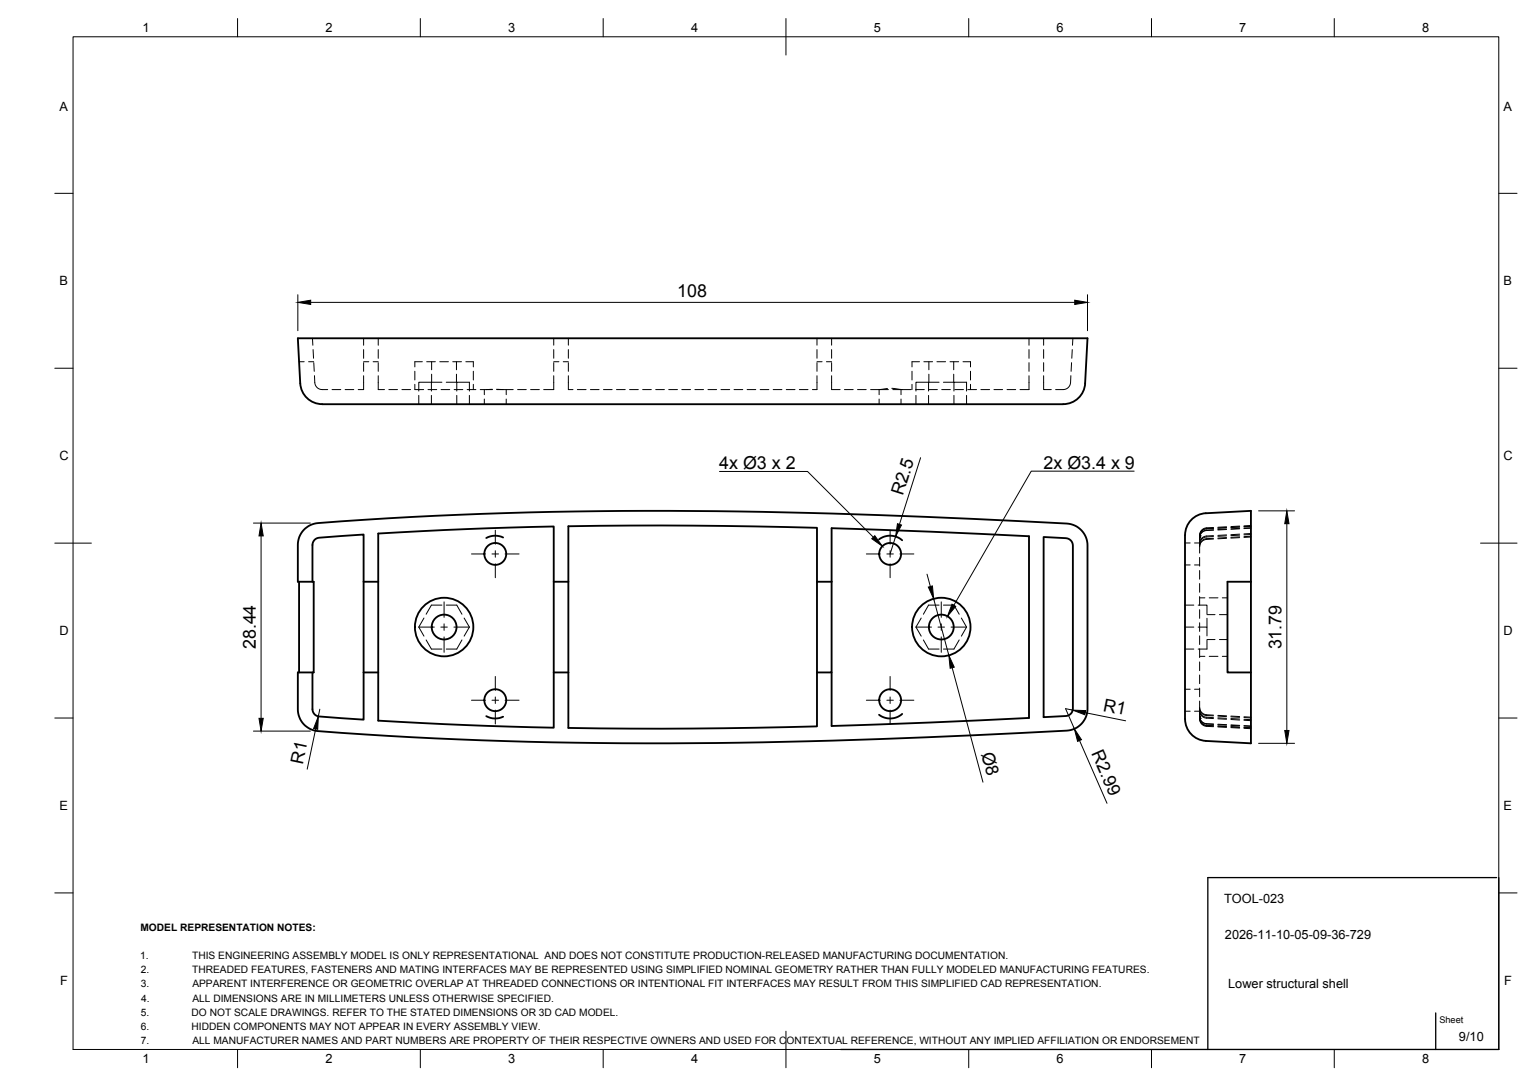
ISO-10303-21;
HEADER;
/* Generated by software containing ST-Developer
 * from STEP Tools, Inc. (www.steptools.com) 
 */

FILE_DESCRIPTION(
/* description */ (''),
/* implementation_level */ '2;1');

FILE_NAME(
/* name */ 'Lower structural shell.step',
/* time_stamp */ '2026-11-10T05:40:20-08:00',
/* author */ (''),
/* organization */ (''),
/* preprocessor_version */ 'ST-DEVELOPER v20.2',
/* originating_system */ 'Autodesk Translation Framework v15.17.0.0',
/* authorisation */ '');

FILE_SCHEMA (('AUTOMOTIVE_DESIGN { 1 0 10303 214 3 1 1 }'));
ENDSEC;

DATA;
#10=MECHANICAL_DESIGN_GEOMETRIC_PRESENTATION_REPRESENTATION('',(#576),#18580);
#84=SPHERICAL_SURFACE('',#6911,0.1);
#85=SPHERICAL_SURFACE('',#6914,0.0999999999999998);
#86=SPHERICAL_SURFACE('',#6918,0.0999999999999993);
#87=SPHERICAL_SURFACE('',#6922,0.1);
#88=SPHERICAL_SURFACE('',#6927,0.3);
#89=SPHERICAL_SURFACE('',#6931,0.3);
#90=SPHERICAL_SURFACE('',#6935,0.299999999999999);
#91=SPHERICAL_SURFACE('',#6940,0.3);
#124=B_SPLINE_SURFACE_WITH_KNOTS('',3,3,((#10861,#10862,#10863,#10864),
(#10865,#10866,#10867,#10868),(#10869,#10870,#10871,#10872),(#10873,#10874,
#10875,#10876),(#10877,#10878,#10879,#10880)),.UNSPECIFIED.,.F.,.F.,.F.,
(4,1,4),(4,4),(0.,0.571428571428571,1.),(1.0454440030657,3.44967454744645),
 .UNSPECIFIED.);
#125=B_SPLINE_SURFACE_WITH_KNOTS('',3,3,((#10953,#10954,#10955,#10956),
(#10957,#10958,#10959,#10960),(#10961,#10962,#10963,#10964),(#10965,#10966,
#10967,#10968),(#10969,#10970,#10971,#10972)),.UNSPECIFIED.,.F.,.F.,.F.,
(4,1,4),(4,4),(0.,0.571428571428571,1.),(7.24519303641511,9.95046872158573),
 .UNSPECIFIED.);
#126=B_SPLINE_SURFACE_WITH_KNOTS('',3,3,((#11894,#11895,#11896,#11897),
(#11898,#11899,#11900,#11901),(#11902,#11903,#11904,#11905),(#11906,#11907,
#11908,#11909)),.UNSPECIFIED.,.F.,.F.,.F.,(4,4),(4,4),(0.0705535719740953,
0.323522444336189),(0.0117434863834119,0.684857763552191),.UNSPECIFIED.);
#127=B_SPLINE_SURFACE_WITH_KNOTS('',3,3,((#11914,#11915,#11916,#11917),
(#11918,#11919,#11920,#11921),(#11922,#11923,#11924,#11925),(#11926,#11927,
#11928,#11929)),.UNSPECIFIED.,.F.,.F.,.F.,(4,4),(4,4),(0.0262419052680539,
0.0545428296147404),(0.0121538053864343,0.684980602226481),
 .UNSPECIFIED.);
#128=B_SPLINE_SURFACE_WITH_KNOTS('',3,3,((#11939,#11940,#11941,#11942),
(#11943,#11944,#11945,#11946),(#11947,#11948,#11949,#11950),(#11951,#11952,
#11953,#11954),(#11955,#11956,#11957,#11958)),.UNSPECIFIED.,.F.,.F.,.F.,
(4,1,4),(4,4),(0.,0.571428571428571,1.),(0.752061768057538,3.45733745322815),
 .UNSPECIFIED.);
#129=B_SPLINE_SURFACE_WITH_KNOTS('',3,3,((#11959,#11960,#11961,#11962),
(#11963,#11964,#11965,#11966),(#11967,#11968,#11969,#11970),(#11971,#11972,
#11973,#11974),(#11975,#11976,#11977,#11978)),.UNSPECIFIED.,.F.,.F.,.F.,
(4,1,4),(4,4),(0.,0.571428571428571,1.),(0.283259008618247,0.557056952888827),
 .UNSPECIFIED.);
#130=B_SPLINE_SURFACE_WITH_KNOTS('',3,3,((#11992,#11993,#11994,#11995),
(#11996,#11997,#11998,#11999),(#12000,#12001,#12002,#12003),(#12004,#12005,
#12006,#12007)),.UNSPECIFIED.,.F.,.F.,.F.,(4,4),(4,4),(0.67647755566375,
0.929446428026011),(0.0117434863436937,0.684857763580381),.UNSPECIFIED.);
#131=B_SPLINE_SURFACE_WITH_KNOTS('',3,3,((#12008,#12009,#12010,#12011),
(#12012,#12013,#12014,#12015),(#12016,#12017,#12018,#12019),(#12020,#12021,
#12022,#12023)),.UNSPECIFIED.,.F.,.F.,.F.,(4,4),(4,4),(0.945457170385156,
0.973758094731946),(0.0121538053598088,0.684980602226481),.UNSPECIFIED.);
#132=B_SPLINE_SURFACE_WITH_KNOTS('',3,3,((#12107,#12108,#12109,#12110),
(#12111,#12112,#12113,#12114),(#12115,#12116,#12117,#12118),(#12119,#12120,
#12121,#12122)),.UNSPECIFIED.,.F.,.F.,.F.,(4,4),(4,4),(0.341142793678372,
0.658675488550287),(0.0116221239297273,0.684255166525269),.UNSPECIFIED.);
#133=B_SPLINE_SURFACE_WITH_KNOTS('',3,3,((#12127,#12128,#12129,#12130),
(#12131,#12132,#12133,#12134),(#12135,#12136,#12137,#12138),(#12139,#12140,
#12141,#12142),(#12143,#12144,#12145,#12146)),.UNSPECIFIED.,.F.,.F.,.F.,
(4,1,4),(4,4),(0.,0.571428571428571,1.),(3.65450559744172,7.0548588409572),
 .UNSPECIFIED.);
#134=B_SPLINE_SURFACE_WITH_KNOTS('',3,3,((#12156,#12157,#12158,#12159),
(#12160,#12161,#12162,#12163),(#12164,#12165,#12166,#12167),(#12168,#12169,
#12170,#12171),(#12172,#12173,#12174,#12175)),.UNSPECIFIED.,.F.,.F.,.F.,
(4,1,4),(4,4),(0.,0.571428571428571,1.),(3.64767164868607,7.04802489220155),
 .UNSPECIFIED.);
#135=B_SPLINE_SURFACE_WITH_KNOTS('',3,3,((#12180,#12181,#12182,#12183),
(#12184,#12185,#12186,#12187),(#12188,#12189,#12190,#12191),(#12192,#12193,
#12194,#12195)),.UNSPECIFIED.,.F.,.F.,.F.,(4,4),(4,4),(0.341324511449716,
0.658857206321627),(0.0116221214776208,0.684255166525269),.UNSPECIFIED.);
#136=B_SPLINE_SURFACE_WITH_KNOTS('',3,3,((#12240,#12241,#12242,#12243),
(#12244,#12245,#12246,#12247),(#12248,#12249,#12250,#12251),(#12252,#12253,
#12254,#12255)),.UNSPECIFIED.,.F.,.F.,.F.,(4,4),(4,4),(0.676316266718331,
0.901708040522105),(0.0117102006467275,0.68495201331719),.UNSPECIFIED.);
#137=B_SPLINE_SURFACE_WITH_KNOTS('',3,3,((#12260,#12261,#12262,#12263),
(#12264,#12265,#12266,#12267),(#12268,#12269,#12270,#12271),(#12272,#12273,
#12274,#12275),(#12276,#12277,#12278,#12279)),.UNSPECIFIED.,.F.,.F.,.F.,
(4,1,4),(4,4),(0.,0.571428571428571,1.),(7.25285594219682,9.65708648657758),
 .UNSPECIFIED.);
#138=B_SPLINE_SURFACE_WITH_KNOTS('',3,3,((#12289,#12290,#12291,#12292),
(#12293,#12294,#12295,#12296),(#12297,#12298,#12299,#12300),(#12301,#12302,
#12303,#12304)),.UNSPECIFIED.,.F.,.F.,.F.,(4,4),(4,4),(0.0982919594778951,
0.323683733281714),(0.0117102006467272,0.68495201331719),.UNSPECIFIED.);
#139=B_SPLINE_SURFACE_WITH_KNOTS('',3,3,((#12379,#12380,#12381,#12382),
(#12383,#12384,#12385,#12386),(#12387,#12388,#12389,#12390),(#12391,#12392,
#12393,#12394)),.UNSPECIFIED.,.F.,.F.,.F.,(4,4),(4,4),(0.917922863855343,
0.974411608827007),(0.0122403473423911,0.685344304754238),.UNSPECIFIED.);
#140=B_SPLINE_SURFACE_WITH_KNOTS('',3,3,((#12404,#12405,#12406,#12407),
(#12408,#12409,#12410,#12411),(#12412,#12413,#12414,#12415),(#12416,#12417,
#12418,#12419),(#12420,#12421,#12422,#12423)),.UNSPECIFIED.,.F.,.F.,.F.,
(4,1,4),(4,4),(0.,0.571428571428571,1.),(9.85085636625011,10.4271318523291),
 .UNSPECIFIED.);
#141=B_SPLINE_SURFACE_WITH_KNOTS('',3,3,((#12437,#12438,#12439,#12440),
(#12441,#12442,#12443,#12444),(#12445,#12446,#12447,#12448),(#12449,#12450,
#12451,#12452)),.UNSPECIFIED.,.F.,.F.,.F.,(4,4),(4,4),(0.025588391172993,
0.0820771361446569),(0.0122403473423911,0.685344304754238),
 .UNSPECIFIED.);
#142=B_SPLINE_SURFACE_WITH_KNOTS('',3,3,((#12462,#12463,#12464,#12465),
(#12466,#12467,#12468,#12469),(#12470,#12471,#12472,#12473),(#12474,#12475,
#12476,#12477),(#12478,#12479,#12480,#12481)),.UNSPECIFIED.,.F.,.F.,.F.,
(4,1,4),(4,4),(0.,0.571428571428571,1.),(0.27539863731415,0.851674123393175),
 .UNSPECIFIED.);
#143=B_SPLINE_SURFACE_WITH_KNOTS('',3,3,((#12495,#12496,#12497,#12498),
(#12499,#12500,#12501,#12502),(#12503,#12504,#12505,#12506),(#12507,#12508,
#12509,#12510),(#12511,#12512,#12513,#12514)),.UNSPECIFIED.,.F.,.F.,.F.,
(4,1,4),(4,4),(0.,0.571428571428571,1.),(0.00944995813270487,0.618489359031386),
 .UNSPECIFIED.);
#144=B_SPLINE_SURFACE_WITH_KNOTS('',3,3,((#12521,#12522,#12523,#12524),
(#12525,#12526,#12527,#12528),(#12529,#12530,#12531,#12532),(#12533,#12534,
#12535,#12536),(#12537,#12538,#12539,#12540)),.UNSPECIFIED.,.F.,.F.,.F.,
(4,1,4),(4,4),(0.,0.571428571428571,1.),(0.00908570715245136,0.618164468641375),
 .UNSPECIFIED.);
#145=B_SPLINE_SURFACE_WITH_KNOTS('',3,3,((#12545,#12546,#12547,#12548),
(#12549,#12550,#12551,#12552),(#12553,#12554,#12555,#12556),(#12557,#12558,
#12559,#12560),(#12561,#12562,#12563,#12564)),.UNSPECIFIED.,.F.,.F.,.F.,
(4,1,4),(4,4),(0.,0.571428571428571,1.),(0.0091183540525243,0.618164468641375),
 .UNSPECIFIED.);
#146=B_SPLINE_SURFACE_WITH_KNOTS('',3,3,((#12569,#12570,#12571,#12572),
(#12573,#12574,#12575,#12576),(#12577,#12578,#12579,#12580),(#12581,#12582,
#12583,#12584),(#12585,#12586,#12587,#12588)),.UNSPECIFIED.,.F.,.F.,.F.,
(4,1,4),(4,4),(0.,0.571428571428571,1.),(10.1454735367545,10.419271481025),
 .UNSPECIFIED.);
#147=B_SPLINE_SURFACE_WITH_KNOTS('',3,3,((#12589,#12590,#12591,#12592),
(#12593,#12594,#12595,#12596),(#12597,#12598,#12599,#12600),(#12601,#12602,
#12603,#12604),(#12605,#12606,#12607,#12608)),.UNSPECIFIED.,.F.,.F.,.F.,
(4,1,4),(4,4),(0.,0.571428571428571,1.),(0.0094045468285345,0.618489359031386),
 .UNSPECIFIED.);
#148=B_SPLINE_SURFACE_WITH_KNOTS('',3,3,((#12634,#12635,#12636,#12637),
(#12638,#12639,#12640,#12641),(#12642,#12643,#12644,#12645),(#12646,#12647,
#12648,#12649),(#12650,#12651,#12652,#12653)),.UNSPECIFIED.,.F.,.F.,.F.,
(4,1,4),(4,4),(0.,0.571428571428571,1.),(-0.00535061636073277,0.618489359031386),
 .UNSPECIFIED.);
#149=B_SPLINE_SURFACE_WITH_KNOTS('',3,3,((#12672,#12673,#12674,#12675,#12676),
(#12677,#12678,#12679,#12680,#12681),(#12682,#12683,#12684,#12685,#12686),
(#12687,#12688,#12689,#12690,#12691),(#12692,#12693,#12694,#12695,#12696)),
 .UNSPECIFIED.,.F.,.F.,.F.,(4,1,4),(4,1,4),(0.,0.571428571428571,1.),(0.283259008618247,
4.63063308449434,10.4271318523291),.UNSPECIFIED.);
#150=B_SPLINE_SURFACE_WITH_KNOTS('',3,3,((#12707,#12708,#12709,#12710),
(#12711,#12712,#12713,#12714),(#12715,#12716,#12717,#12718),(#12719,#12720,
#12721,#12722),(#12723,#12724,#12725,#12726)),.UNSPECIFIED.,.F.,.F.,.F.,
(4,1,4),(4,4),(0.,0.571428571428571,1.),(-0.00578978989683084,0.618164468641375),
 .UNSPECIFIED.);
#151=B_SPLINE_SURFACE_WITH_KNOTS('',3,3,((#12735,#12736,#12737,#12738),
(#12739,#12740,#12741,#12742),(#12743,#12744,#12745,#12746),(#12747,#12748,
#12749,#12750),(#12751,#12752,#12753,#12754)),.UNSPECIFIED.,.F.,.F.,.F.,
(4,1,4),(4,4),(0.,0.571428571428571,1.),(-0.00569189159989896,0.618164468641375),
 .UNSPECIFIED.);
#152=B_SPLINE_SURFACE_WITH_KNOTS('',3,3,((#12763,#12764,#12765,#12766,#12767),
(#12768,#12769,#12770,#12771,#12772),(#12773,#12774,#12775,#12776,#12777),
(#12778,#12779,#12780,#12781,#12782),(#12783,#12784,#12785,#12786,#12787)),
 .UNSPECIFIED.,.F.,.F.,.F.,(4,1,4),(4,1,4),(0.,0.571428571428571,1.),(0.27539863731415,
4.62277271319024,10.419271481025),.UNSPECIFIED.);
#153=B_SPLINE_SURFACE_WITH_KNOTS('',3,3,((#12798,#12799,#12800,#12801),
(#12802,#12803,#12804,#12805),(#12806,#12807,#12808,#12809),(#12810,#12811,
#12812,#12813),(#12814,#12815,#12816,#12817)),.UNSPECIFIED.,.F.,.F.,.F.,
(4,1,4),(4,4),(0.,0.571428571428571,1.),(-0.0054868135546625,0.618489359031386),
 .UNSPECIFIED.);
#154=B_SPLINE_SURFACE_WITH_KNOTS('',3,3,((#12826,#12827,#12828,#12829),
(#12830,#12831,#12832,#12833),(#12834,#12835,#12836,#12837),(#12838,#12839,
#12840,#12841)),.UNSPECIFIED.,.F.,.F.,.F.,(4,4),(4,4),(0.026239262514127,
0.974414173651419),(0.,0.685344304754238),.UNSPECIFIED.);
#155=B_SPLINE_SURFACE_WITH_KNOTS('',3,3,((#12844,#12845,#12846,#12847),
(#12848,#12849,#12850,#12851),(#12852,#12853,#12854,#12855),(#12856,#12857,
#12858,#12859)),.UNSPECIFIED.,.F.,.F.,.F.,(4,4),(4,4),(0.0255858263485814,
0.973760737485873),(0.,0.685344304754238),.UNSPECIFIED.);
#272=B_SPLINE_CURVE_WITH_KNOTS('',3,(#10760,#10761,#10762,#10763,#10764,
#10765,#10766,#10767,#10768,#10769,#10770,#10771,#10772,#10773,#10774,#10775,
#10776,#10777,#10778,#10779,#10780,#10781,#10782,#10783),.UNSPECIFIED.,
 .F.,.F.,(4,2,2,2,2,2,2,2,2,2,2,4),(-0.337265338267783,-0.250544943628509,
-0.208272806508042,-0.186542211788094,-0.176382978682897,-0.170925844043069,
-0.16639450677335,-0.161077381235501,-0.15182241135393,-0.115009181549223,
-0.030206004227969,0.),.UNSPECIFIED.);
#273=B_SPLINE_CURVE_WITH_KNOTS('',3,(#10788,#10789,#10790,#10791,#10792,
#10793,#10794,#10795,#10796,#10797,#10798,#10799,#10800,#10801,#10802,#10803,
#10804,#10805,#10806,#10807),.UNSPECIFIED.,.F.,.F.,(4,2,2,2,2,2,2,2,2,4),
(-0.240982594686416,-0.16829976149504,-0.141836598208813,-0.129116059226128,
-0.121962912034391,-0.115857591426886,-0.108506552485159,-0.0948769875819265,
-0.0364654790774683,0.),.UNSPECIFIED.);
#274=B_SPLINE_CURVE_WITH_KNOTS('',3,(#10812,#10813,#10814,#10815,#10816,
#10817,#10818,#10819,#10820,#10821,#10822,#10823,#10824,#10825,#10826,#10827,
#10828,#10829,#10830,#10831),.UNSPECIFIED.,.F.,.F.,(4,2,2,2,2,2,2,2,2,4),
(-0.240981214998207,-0.168303541671295,-0.141841407502325,-0.129121097580905,
-0.121968013294536,-0.115862708924237,-0.108511643765797,-0.0948818976588229,
-0.0364681276985956,0.),.UNSPECIFIED.);
#275=B_SPLINE_CURVE_WITH_KNOTS('',3,(#10836,#10837,#10838,#10839,#10840,
#10841,#10842,#10843,#10844,#10845,#10846,#10847,#10848,#10849,#10850,#10851,
#10852,#10853,#10854,#10855,#10856,#10857,#10858,#10859),.UNSPECIFIED.,
 .F.,.F.,(4,2,2,2,2,2,2,2,2,2,2,4),(-0.337269388373684,-0.250545316912909,
-0.208282401844766,-0.186554569827561,-0.176396213396297,-0.17093921790305,
-0.16640782243471,-0.161090427650893,-0.151834477986603,-0.115010808423941,
-0.0302102096065556,0.),.UNSPECIFIED.);
#276=B_SPLINE_CURVE_WITH_KNOTS('',3,(#10882,#10883,#10884,#10885),
 .UNSPECIFIED.,.F.,.F.,(4,4),(1.0454440030657,2.52465537163019),
 .UNSPECIFIED.);
#277=B_SPLINE_CURVE_WITH_KNOTS('',3,(#10887,#10888,#10889,#10890,#10891,
#10892,#10893,#10894,#10895,#10896,#10897,#10898,#10899,#10900,#10901,#10902,
#10903,#10904,#10905,#10906,#10907,#10908,#10909,#10910,#10911,#10912,#10913,
#10914),.UNSPECIFIED.,.F.,.F.,(4,3,3,3,3,3,3,3,3,4),(-0.152193408756968,
-0.128427023368412,-0.115107736263918,-0.0911810900745799,-0.0780377802127556,
-0.0652031397886901,-0.0414031558437525,-0.0389949527774582,-0.0152076153333754,
0.),.UNSPECIFIED.);
#278=B_SPLINE_CURVE_WITH_KNOTS('',3,(#10916,#10917,#10918,#10919),
 .UNSPECIFIED.,.F.,.F.,(4,4),(-3.44967454744645,-1.05170160817356),
 .UNSPECIFIED.);
#279=B_SPLINE_CURVE_WITH_KNOTS('',3,(#10921,#10922,#10923,#10924,#10925,
#10926,#10927,#10928,#10929,#10930,#10931,#10932,#10933,#10934,#10935,#10936,
#10937,#10938,#10939,#10940,#10941,#10942,#10943,#10944,#10945,#10946,#10947,
#10948),.UNSPECIFIED.,.F.,.F.,(4,3,3,3,3,3,3,3,3,4),(-0.152278960443096,
-0.128503570101575,-0.115218572146868,-0.09145408274965,-0.0870214650669139,
-0.0781562978024333,-0.0542566895399357,-0.03908030849237,-0.0153296112319379,
0.),.UNSPECIFIED.);
#280=B_SPLINE_CURVE_WITH_KNOTS('',3,(#10949,#10950,#10951,#10952),
 .UNSPECIFIED.,.F.,.F.,(4,4),(2.75501813708031,3.4476340663212),
 .UNSPECIFIED.);
#281=B_SPLINE_CURVE_WITH_KNOTS('',3,(#10974,#10975,#10976,#10977),
 .UNSPECIFIED.,.F.,.F.,(4,4),(7.24810383506675,7.89761558728778),
 .UNSPECIFIED.);
#282=B_SPLINE_CURVE_WITH_KNOTS('',3,(#10979,#10980,#10981,#10982,#10983,
#10984,#10985,#10986,#10987,#10988,#10989,#10990,#10991,#10992,#10993,#10994,
#10995,#10996,#10997,#10998,#10999,#11000,#11001,#11002,#11003,#11004,#11005,
#11006),.UNSPECIFIED.,.F.,.F.,(4,3,3,3,3,3,3,3,3,4),(-0.152278869104567,
-0.128548794904564,-0.115192257893812,-0.0912773536606376,-0.0781090575823055,
-0.0652724057916263,-0.0414819581560496,-0.0390493575290778,-0.015259721743698,
0.),.UNSPECIFIED.);
#283=B_SPLINE_CURVE_WITH_KNOTS('',3,(#11008,#11009,#11010,#11011),
 .UNSPECIFIED.,.F.,.F.,(4,4),(-9.94532343034734,-7.24519303641511),
 .UNSPECIFIED.);
#284=B_SPLINE_CURVE_WITH_KNOTS('',3,(#11013,#11014,#11015,#11016,#11017,
#11018,#11019,#11020,#11021,#11022,#11023,#11024,#11025,#11026,#11027,#11028,
#11029,#11030,#11031,#11032,#11033,#11034,#11035,#11036,#11037,#11038,#11039,
#11040),.UNSPECIFIED.,.F.,.F.,(4,3,3,3,3,3,3,3,3,4),(-0.152181623618259,
-0.128410404494075,-0.115248188224843,-0.0914746846046984,-0.0869904866333268,
-0.0783028696190655,-0.0543945376065823,-0.0391651209697638,-0.0153884182770307,
0.),.UNSPECIFIED.);
#285=B_SPLINE_CURVE_WITH_KNOTS('',3,(#11041,#11042,#11043,#11044),
 .UNSPECIFIED.,.F.,.F.,(4,4),(8.21380824320284,9.95046871680089),
 .UNSPECIFIED.);
#286=B_SPLINE_CURVE_WITH_KNOTS('',3,(#11047,#11048,#11049,#11050),
 .UNSPECIFIED.,.F.,.F.,(4,4),(2.80491490332713,3.45442665446657),
 .UNSPECIFIED.);
#287=B_SPLINE_CURVE_WITH_KNOTS('',3,(#11054,#11055,#11056,#11057),
 .UNSPECIFIED.,.F.,.F.,(4,4),(0.752061768057538,2.48872224644044),
 .UNSPECIFIED.);
#288=B_SPLINE_CURVE_WITH_KNOTS('',3,(#11265,#11266,#11267,#11268,#11269,
#11270),.UNSPECIFIED.,.F.,.F.,(4,2,4),(-0.606700505977711,-0.303383635264422,
-0.000339350725729326),.UNSPECIFIED.);
#289=B_SPLINE_CURVE_WITH_KNOTS('',3,(#11271,#11272,#11273,#11274,#11275,
#11276,#11277,#11278,#11279,#11280,#11281,#11282,#11283,#11284,#11285,#11286,
#11287,#11288,#11289,#11290,#11291,#11292,#11293,#11294,#11295,#11296,#11297,
#11298),.UNSPECIFIED.,.F.,.F.,(4,3,3,3,3,3,3,3,3,4),(-0.152173579228948,
-0.128423230539522,-0.115115104157663,-0.0911927259648815,-0.0780672068328041,
-0.0652082609452843,-0.0414117413801899,-0.0390174000215468,-0.0152300060615686,
0.),.UNSPECIFIED.);
#290=B_SPLINE_CURVE_WITH_KNOTS('',3,(#11299,#11300,#11301,#11302,#11303,
#11304),.UNSPECIFIED.,.F.,.F.,(4,2,4),(-0.606471894652381,-0.303383500305553,
-0.00011071898471493),.UNSPECIFIED.);
#291=B_SPLINE_CURVE_WITH_KNOTS('',3,(#11308,#11309,#11310,#11311,#11312,
#11313),.UNSPECIFIED.,.F.,.F.,(4,2,4),(-0.606240625011114,-0.303433113375332,
-0.00010938105916114),.UNSPECIFIED.);
#292=B_SPLINE_CURVE_WITH_KNOTS('',3,(#11315,#11316,#11317,#11318,#11319,
#11320,#11321,#11322,#11323,#11324,#11325,#11326,#11327,#11328,#11329,#11330,
#11331,#11332,#11333,#11334,#11335,#11336,#11337,#11338,#11339,#11340,#11341,
#11342),.UNSPECIFIED.,.F.,.F.,(4,3,3,3,3,3,3,3,3,4),(-0.152281454644235,
-0.128508102092242,-0.115234945630277,-0.0914677943501604,-0.0870276017853555,
-0.0781846052914712,-0.0542821334115454,-0.0390966859411886,-0.0153419673568312,
0.),.UNSPECIFIED.);
#293=B_SPLINE_CURVE_WITH_KNOTS('',3,(#11344,#11345,#11346,#11347,#11348,
#11349),.UNSPECIFIED.,.F.,.F.,(4,2,4),(-0.606758573154242,-0.303433157101101,
-0.000627306481538803),.UNSPECIFIED.);
#294=B_SPLINE_CURVE_WITH_KNOTS('',3,(#11355,#11356,#11357,#11358,#11359,
#11360),.UNSPECIFIED.,.F.,.F.,(4,2,4),(-0.60617382748,-0.303436117212405,
-7.2700296824213E-5),.UNSPECIFIED.);
#295=B_SPLINE_CURVE_WITH_KNOTS('',3,(#11362,#11363,#11364,#11365,#11366,
#11367,#11368,#11369,#11370,#11371,#11372,#11373,#11374,#11375,#11376,#11377,
#11378,#11379,#11380,#11381,#11382,#11383,#11384,#11385,#11386,#11387,#11388,
#11389),.UNSPECIFIED.,.F.,.F.,(4,3,3,3,3,3,3,3,3,4),(-0.152282154327755,
-0.128558036203745,-0.115201429639692,-0.0912891813973639,-0.0781219052297615,
-0.065279687589213,-0.0414913146723999,-0.0390591331507366,-0.0152683745546824,
0.),.UNSPECIFIED.);
#296=B_SPLINE_CURVE_WITH_KNOTS('',3,(#11393,#11394,#11395,#11396,#11397,
#11398,#11399,#11400,#11401,#11402,#11403,#11404,#11405,#11406,#11407,#11408,
#11409,#11410,#11411,#11412,#11413,#11414,#11415,#11416,#11417,#11418,#11419,
#11420),.UNSPECIFIED.,.F.,.F.,(4,3,3,3,3,3,3,3,3,4),(-0.152283066055976,
-0.128508717930245,-0.115216472798554,-0.091451700383826,-0.087022506454752,
-0.0781485278686168,-0.0542483994686567,-0.0390758108455304,-0.0153274175274101,
0.),.UNSPECIFIED.);
#297=B_SPLINE_CURVE_WITH_KNOTS('',3,(#11422,#11423,#11424,#11425,#11426,
#11427),.UNSPECIFIED.,.F.,.F.,(4,2,4),(-0.606800264911061,-0.303436147592132,
-0.000699137727853738),.UNSPECIFIED.);
#298=B_SPLINE_CURVE_WITH_KNOTS('',3,(#11432,#11433,#11434,#11435,#11436,
#11437),.UNSPECIFIED.,.F.,.F.,(4,2,4),(-0.606915279655722,-0.30363236403835,
-0.000516487074480598),.UNSPECIFIED.);
#299=B_SPLINE_CURVE_WITH_KNOTS('',3,(#11441,#11442,#11443,#11444,#11445,
#11446,#11447,#11448,#11449,#11450,#11451,#11452,#11453,#11454,#11455,#11456,
#11457,#11458,#11459,#11460,#11461,#11462,#11463,#11464,#11465,#11466,#11467,
#11468),.UNSPECIFIED.,.F.,.F.,(4,3,3,3,3,3,3,3,3,4),(-0.152205325335401,
-0.128433618138404,-0.115304790388008,-0.091527299141506,-0.0870178586418932,
-0.0783866443643876,-0.0544751548276533,-0.0392137310602028,-0.0154203878854647,
0.),.UNSPECIFIED.);
#300=B_SPLINE_CURVE_WITH_KNOTS('',3,(#11470,#11471,#11472,#11473,#11474,
#11475),.UNSPECIFIED.,.F.,.F.,(4,2,4),(-0.606752424187958,-0.303632696349781,
-0.000353591088346872),.UNSPECIFIED.);
#301=B_SPLINE_CURVE_WITH_KNOTS('',3,(#11481,#11482,#11483,#11484),
 .UNSPECIFIED.,.F.,.F.,(4,4),(0.0116023361771303,0.618489359031386),
 .UNSPECIFIED.);
#302=B_SPLINE_CURVE_WITH_KNOTS('',3,(#11488,#11489,#11490,#11491),
 .UNSPECIFIED.,.F.,.F.,(4,4),(-0.618489359031386,-0.01160233617713),
 .UNSPECIFIED.);
#303=B_SPLINE_CURVE_WITH_KNOTS('',3,(#11494,#11495,#11496,#11497),
 .UNSPECIFIED.,.F.,.F.,(4,4),(7.01593971618694,9.71770560667459),
 .UNSPECIFIED.);
#304=B_SPLINE_CURVE_WITH_KNOTS('',3,(#11498,#11499,#11500,#11501),
 .UNSPECIFIED.,.F.,.F.,(4,4),(0.505945342046796,3.20718651982575),
 .UNSPECIFIED.);
#305=B_SPLINE_CURVE_WITH_KNOTS('',3,(#11504,#11505,#11506,#11507,#11508,
#11509,#11510),.UNSPECIFIED.,.F.,.F.,(4,3,4),(3.40717417387402,5.11170895874517,
6.80746068626633),.UNSPECIFIED.);
#306=B_SPLINE_CURVE_WITH_KNOTS('',3,(#11513,#11514,#11515,#11516),
 .UNSPECIFIED.,.F.,.F.,(4,4),(7.00766573366377,9.41198845520559),
 .UNSPECIFIED.);
#307=B_SPLINE_CURVE_WITH_KNOTS('',3,(#11520,#11521,#11522,#11523),
 .UNSPECIFIED.,.F.,.F.,(4,4),(9.61248784142317,10.2217363065808),
 .UNSPECIFIED.);
#308=B_SPLINE_CURVE_WITH_KNOTS('',3,(#11524,#11525,#11526,#11527,#11528,
#11529,#11530,#11531,#11532,#11533,#11534,#11535,#11536,#11537,#11538,#11539,
#11540,#11541,#11542,#11543,#11544,#11545,#11546,#11547,#11548,#11549,#11550,
#11551),.UNSPECIFIED.,.F.,.F.,(4,3,3,3,3,3,3,3,3,4),(0.,0.0238103109064959,
0.0390781362249314,0.0628635086275546,0.0641230352384255,0.0780643700703951,
0.101962174814111,0.113803522271848,0.137549611554782,0.149564734365165),
 .UNSPECIFIED.);
#309=B_SPLINE_CURVE_WITH_KNOTS('',3,(#11555,#11556,#11557,#11558,#11559,
#11560,#11561,#11562,#11563,#11564,#11565,#11566,#11567,#11568,#11569,#11570,
#11571,#11572,#11573,#11574,#11575,#11576,#11577,#11578,#11579,#11580,#11581,
#11582,#11583,#11584,#11585),.UNSPECIFIED.,.F.,.F.,(4,3,3,3,3,3,3,3,3,3,
4),(0.,0.0535521515156599,0.107729685495911,0.117233338918226,0.171447998942947,
0.1923696899792,0.234191611538245,0.288659693466396,0.341410301570312,0.395549383747909,
0.448696573746633),.UNSPECIFIED.);
#310=B_SPLINE_CURVE_WITH_KNOTS('',3,(#11587,#11588,#11589,#11590),
 .UNSPECIFIED.,.F.,.F.,(4,4),(0.0255858263485814,0.973760737485873),
 .UNSPECIFIED.);
#311=B_SPLINE_CURVE_WITH_KNOTS('',3,(#11592,#11593,#11594,#11595,#11596,
#11597,#11598,#11599,#11600,#11601,#11602,#11603,#11604,#11605,#11606,#11607,
#11608,#11609,#11610,#11611,#11612,#11613,#11614,#11615,#11616,#11617,#11618,
#11619,#11620,#11621,#11622),.UNSPECIFIED.,.F.,.F.,(4,3,3,3,3,3,3,3,3,3,
4),(0.,0.0535144560117858,0.107726856902975,0.117300577410231,0.171517675930231,
0.195438847090422,0.234297456941738,0.289665153342662,0.345032849743585,
0.40043206955427,0.455831289364955),.UNSPECIFIED.);
#312=B_SPLINE_CURVE_WITH_KNOTS('',3,(#11626,#11627,#11628,#11629,#11630,
#11631,#11632,#11633,#11634,#11635,#11636,#11637,#11638,#11639,#11640,#11641,
#11642,#11643,#11644,#11645,#11646,#11647,#11648,#11649,#11650,#11651,#11652,
#11653,#11654,#11655,#11656),.UNSPECIFIED.,.F.,.F.,(4,3,3,3,3,3,3,3,3,3,
4),(0.,0.053505543180391,0.107714168832353,0.117253997025819,0.171473395203321,
0.195418854185489,0.234223199196375,0.289607016015183,0.344990832833991,
0.400409777473312,0.455828722112633),.UNSPECIFIED.);
#313=B_SPLINE_CURVE_WITH_KNOTS('',3,(#11658,#11659,#11660,#11661),
 .UNSPECIFIED.,.F.,.F.,(4,4),(0.0262392625141271,0.974414173651419),
 .UNSPECIFIED.);
#314=B_SPLINE_CURVE_WITH_KNOTS('',3,(#11663,#11664,#11665,#11666,#11667,
#11668,#11669,#11670,#11671,#11672,#11673,#11674,#11675,#11676,#11677,#11678,
#11679,#11680,#11681,#11682,#11683,#11684,#11685,#11686,#11687,#11688,#11689,
#11690,#11691,#11692,#11693),.UNSPECIFIED.,.F.,.F.,(4,3,3,3,3,3,3,3,3,3,
4),(0.,0.0535648734523888,0.107747221190676,0.117299947751206,0.171510987106922,
0.192397607227928,0.234296687348373,0.288768001369001,0.341469499352622,
0.395597672314973,0.448700135162036),.UNSPECIFIED.);
#315=B_SPLINE_CURVE_WITH_KNOTS('',3,(#11696,#11697,#11698,#11699,#11700,
#11701,#11702,#11703,#11704,#11705,#11706,#11707,#11708,#11709,#11710,#11711,
#11712,#11713,#11714,#11715,#11716,#11717,#11718,#11719,#11720),
 .UNSPECIFIED.,.F.,.F.,(4,3,3,3,3,3,3,3,4),(0.,0.0238141989470671,0.0391004231578824,
0.0641320992313133,0.0780996136084711,0.101998806889826,0.113823260594808,
0.137564745199532,0.149565921982294),.UNSPECIFIED.);
#316=B_SPLINE_CURVE_WITH_KNOTS('',3,(#11722,#11723,#11724,#11725),
 .UNSPECIFIED.,.F.,.F.,(4,4),(2.76692059912875E-5,0.609394470571143),
 .UNSPECIFIED.);
#317=B_SPLINE_CURVE_WITH_KNOTS('',3,(#11728,#11729,#11730,#11731),
 .UNSPECIFIED.,.F.,.F.,(4,4),(0.809932799154201,3.21472245120952),
 .UNSPECIFIED.);
#318=B_SPLINE_CURVE_WITH_KNOTS('',3,(#11734,#11735,#11736,#11737,#11738,
#11739,#11740),.UNSPECIFIED.,.F.,.F.,(4,3,4),(3.41496637450242,5.11093193409745,
6.81591321610411),.UNSPECIFIED.);
#319=B_SPLINE_CURVE_WITH_KNOTS('',3,(#11744,#11745,#11746,#11747),
 .UNSPECIFIED.,.F.,.F.,(4,4),(9.91798263530139,10.2237206759544),
 .UNSPECIFIED.);
#320=B_SPLINE_CURVE_WITH_KNOTS('',3,(#11749,#11750,#11751,#11752,#11753,
#11754,#11755,#11756,#11757,#11758,#11759,#11760,#11761,#11762,#11763,#11764,
#11765,#11766,#11767,#11768,#11769,#11770,#11771,#11772,#11773,#11774,#11775,
#11776),.UNSPECIFIED.,.F.,.F.,(4,3,3,3,3,3,3,3,3,4),(0.,0.023807020713713,
0.039085080816122,0.0628703378723092,0.0651394887354207,0.0780750047750988,
0.101981498769656,0.114997221725907,0.138748569029605,0.151942344104828),
 .UNSPECIFIED.);
#321=B_SPLINE_CURVE_WITH_KNOTS('',3,(#11780,#11781,#11782,#11783,#11784,
#11785,#11786,#11787,#11788,#11789,#11790,#11791,#11792,#11793,#11794,#11795,
#11796,#11797,#11798,#11799,#11800,#11801,#11802,#11803,#11804,#11805,#11806,
#11807),.UNSPECIFIED.,.F.,.F.,(4,3,3,3,3,3,3,3,3,4),(0.,0.0238098191818892,
0.0391006681981376,0.0628849269680955,0.0651459659463291,0.0780999162396042,
0.102007524384594,0.115011225379555,0.138759376430353,0.151943200125079),
 .UNSPECIFIED.);
#322=B_SPLINE_CURVE_WITH_KNOTS('',3,(#11809,#11810,#11811,#11812),
 .UNSPECIFIED.,.F.,.F.,(4,4),(2.85486020485948E-5,0.305707210239178),
 .UNSPECIFIED.);
#323=B_SPLINE_CURVE_WITH_KNOTS('',3,(#11822,#11823,#11824,#11825,#11826,
#11827),.UNSPECIFIED.,.F.,.F.,(4,2,4),(-0.606446248197249,-0.303383959626182,
-6.4365448350312E-5),.UNSPECIFIED.);
#324=B_SPLINE_CURVE_WITH_KNOTS('',3,(#11829,#11830,#11831,#11832,#11833,
#11834),.UNSPECIFIED.,.F.,.F.,(4,2,4),(-0.60675170080159,-0.303384112192838,
-0.000369837888147484),.UNSPECIFIED.);
#325=B_SPLINE_CURVE_WITH_KNOTS('',3,(#11836,#11837,#11838,#11839,#11840,
#11841,#11842,#11843,#11844,#11845,#11846,#11847,#11848,#11849,#11850,#11851,
#11852,#11853,#11854,#11855,#11856,#11857,#11858,#11859,#11860,#11861,#11862,
#11863),.UNSPECIFIED.,.F.,.F.,(4,3,3,3,3,3,3,3,3,4),(-0.152162866344201,
-0.128411131698784,-0.115108013904405,-0.0911850729173883,-0.0780642464630149,
-0.0652023242402653,-0.0414053499882389,-0.0390151293250392,-0.0152279490549848,
0.),.UNSPECIFIED.);
#326=B_SPLINE_CURVE_WITH_KNOTS('',3,(#11866,#11867,#11868,#11869,#11870,
#11871,#11872,#11873,#11874,#11875,#11876,#11877,#11878,#11879,#11880,#11881,
#11882,#11883,#11884,#11885,#11886,#11887,#11888,#11889,#11890,#11891,#11892,
#11893),.UNSPECIFIED.,.F.,.F.,(4,3,3,3,3,3,3,3,3,4),(-0.152171297476962,
-0.128400300768352,-0.115247520946962,-0.0914735511738372,-0.0869860114952295,
-0.0783112904282795,-0.0544025203706761,-0.0391699941254272,-0.015391764586027,
0.),.UNSPECIFIED.);
#327=B_SPLINE_CURVE_WITH_KNOTS('',3,(#11910,#11911,#11912,#11913),
 .UNSPECIFIED.,.F.,.F.,(4,4),(-3.45733745322815,-0.757207059295936),
 .UNSPECIFIED.);
#328=B_SPLINE_CURVE_WITH_KNOTS('',3,(#11931,#11932,#11933,#11934),
 .UNSPECIFIED.,.F.,.F.,(4,4),(-0.557056952888827,-0.283259008618247),
 .UNSPECIFIED.);
#329=B_SPLINE_CURVE_WITH_KNOTS('',3,(#11935,#11936,#11937,#11938),
 .UNSPECIFIED.,.F.,.F.,(4,4),(-0.618164468641375,-0.0110156167597059),
 .UNSPECIFIED.);
#330=B_SPLINE_CURVE_WITH_KNOTS('',3,(#11980,#11981,#11982,#11983),
 .UNSPECIFIED.,.F.,.F.,(4,4),(0.283259011433088,0.551788488929761),
 .UNSPECIFIED.);
#331=B_SPLINE_CURVE_WITH_KNOTS('',3,(#11987,#11988,#11989,#11990),
 .UNSPECIFIED.,.F.,.F.,(4,4),(10.1507419987596,10.419271481025),
 .UNSPECIFIED.);
#332=B_SPLINE_CURVE_WITH_KNOTS('',3,(#12025,#12026,#12027,#12028),
 .UNSPECIFIED.,.F.,.F.,(4,4),(0.0110156167597055,0.618164468641375),
 .UNSPECIFIED.);
#333=B_SPLINE_CURVE_WITH_KNOTS('',3,(#12029,#12030,#12031,#12032),
 .UNSPECIFIED.,.F.,.F.,(4,4),(-10.419271481025,-10.1454735367545),
 .UNSPECIFIED.);
#334=B_SPLINE_CURVE_WITH_KNOTS('',3,(#12035,#12036,#12037,#12038,#12039,
#12040),.UNSPECIFIED.,.F.,.F.,(4,2,4),(-0.606211482799139,-0.303431960476852,
-9.19895310989571E-5),.UNSPECIFIED.);
#335=B_SPLINE_CURVE_WITH_KNOTS('',3,(#12042,#12043,#12044,#12045,#12046,
#12047,#12048,#12049,#12050,#12051,#12052,#12053,#12054,#12055,#12056,#12057,
#12058,#12059,#12060,#12061,#12062,#12063,#12064,#12065,#12066,#12067,#12068,
#12069),.UNSPECIFIED.,.F.,.F.,(4,3,3,3,3,3,3,3,3,4),(-0.152283340966725,
-0.128554242174982,-0.115196092098682,-0.0912819860997417,-0.0781117853096875,
-0.0652755629514801,-0.0414857317972147,-0.039051434275634,-0.0152612146291672,
0.),.UNSPECIFIED.);
#336=B_SPLINE_CURVE_WITH_KNOTS('',3,(#12073,#12074,#12075,#12076,#12077,
#12078,#12079,#12080,#12081,#12082,#12083,#12084,#12085,#12086,#12087,#12088,
#12089,#12090,#12091,#12092,#12093,#12094,#12095,#12096,#12097,#12098,#12099,
#12100),.UNSPECIFIED.,.F.,.F.,(4,3,3,3,3,3,3,3,3,4),(-0.152285570909379,
-0.128511627155755,-0.115232904621082,-0.0914664612111958,-0.0870286654075453,
-0.0781769338106538,-0.0542752301960614,-0.039092246575741,-0.0153386136911565,
0.),.UNSPECIFIED.);
#337=B_SPLINE_CURVE_WITH_KNOTS('',3,(#12101,#12102,#12103,#12104,#12105,
#12106),.UNSPECIFIED.,.F.,.F.,(4,2,4),(-0.606773318344362,-0.303431998667662,
-0.000653802131222458),.UNSPECIFIED.);
#338=B_SPLINE_CURVE_WITH_KNOTS('',3,(#12123,#12124,#12125,#12126),
 .UNSPECIFIED.,.F.,.F.,(4,4),(-7.05313168653828,-3.6572084986735),
 .UNSPECIFIED.);
#339=B_SPLINE_CURVE_WITH_KNOTS('',3,(#12147,#12148,#12149,#12150),
 .UNSPECIFIED.,.F.,.F.,(4,4),(3.65450559744172,7.0548588409572),
 .UNSPECIFIED.);
#340=B_SPLINE_CURVE_WITH_KNOTS('',3,(#12152,#12153,#12154,#12155),
 .UNSPECIFIED.,.F.,.F.,(4,4),(3.64767164868607,7.04802489220155),
 .UNSPECIFIED.);
#341=B_SPLINE_CURVE_WITH_KNOTS('',3,(#12176,#12177,#12178,#12179),
 .UNSPECIFIED.,.F.,.F.,(4,4),(-7.04532199096977,-3.64939880310499),
 .UNSPECIFIED.);
#342=B_SPLINE_CURVE_WITH_KNOTS('',3,(#12198,#12199,#12200,#12201,#12202,
#12203),.UNSPECIFIED.,.F.,.F.,(4,2,4),(-0.606200453641641,-0.30343602424441,
-9.0120313562092E-5),.UNSPECIFIED.);
#343=B_SPLINE_CURVE_WITH_KNOTS('',3,(#12205,#12206,#12207,#12208,#12209,
#12210,#12211,#12212,#12213,#12214,#12215,#12216,#12217,#12218,#12219,#12220,
#12221,#12222,#12223,#12224,#12225,#12226,#12227,#12228,#12229,#12230,#12231,
#12232),.UNSPECIFIED.,.F.,.F.,(4,3,3,3,3,3,3,3,3,4),(-0.152277688086818,
-0.128551334178815,-0.115197577176818,-0.0912856014461669,-0.0781191417238373,
-0.0652765169533013,-0.0414883027365163,-0.0390570310290822,-0.0152653090895913,
0.),.UNSPECIFIED.);
#344=B_SPLINE_CURVE_WITH_KNOTS('',3,(#12234,#12235,#12236,#12237,#12238,
#12239),.UNSPECIFIED.,.F.,.F.,(4,2,4),(-0.60678286609787,-0.303436074842897,
-0.000672492961417026),.UNSPECIFIED.);
#345=B_SPLINE_CURVE_WITH_KNOTS('',3,(#12256,#12257,#12258,#12259),
 .UNSPECIFIED.,.F.,.F.,(4,4),(-9.65082888146972,-7.25285594219682),
 .UNSPECIFIED.);
#346=B_SPLINE_CURVE_WITH_KNOTS('',3,(#12280,#12281,#12282,#12283),
 .UNSPECIFIED.,.F.,.F.,(4,4),(7.25489642332205,7.94751235889625),
 .UNSPECIFIED.);
#347=B_SPLINE_CURVE_WITH_KNOTS('',3,(#12284,#12285,#12286,#12287),
 .UNSPECIFIED.,.F.,.F.,(4,4),(8.17787511801303,9.65708648657758),
 .UNSPECIFIED.);
#348=B_SPLINE_CURVE_WITH_KNOTS('',3,(#12307,#12308,#12309,#12310,#12311,
#12312),.UNSPECIFIED.,.F.,.F.,(4,2,4),(-0.607007797795788,-0.303636495504298,
-0.000571323176327465),.UNSPECIFIED.);
#349=B_SPLINE_CURVE_WITH_KNOTS('',3,(#12314,#12315,#12316,#12317,#12318,
#12319,#12320,#12321,#12322,#12323,#12324,#12325,#12326,#12327,#12328,#12329,
#12330,#12331,#12332,#12333,#12334,#12335,#12336,#12337,#12338,#12339,#12340,
#12341),.UNSPECIFIED.,.F.,.F.,(4,3,3,3,3,3,3,3,3,4),(-0.152184339020145,
-0.128410461444444,-0.115096394428865,-0.0911692948751363,-0.0780261759644403,
-0.0651939085034322,-0.0413932235702045,-0.0389860720679279,-0.0151971168406065,
0.),.UNSPECIFIED.);
#350=B_SPLINE_CURVE_WITH_KNOTS('',3,(#12345,#12346,#12347,#12348,#12349,
#12350,#12351,#12352,#12353,#12354,#12355,#12356,#12357,#12358,#12359,#12360,
#12361,#12362,#12363,#12364,#12365,#12366,#12367,#12368,#12369,#12370,#12371,
#12372),.UNSPECIFIED.,.F.,.F.,(4,3,3,3,3,3,3,3,3,4),(-0.15219777746951,
-0.128424216118147,-0.115318679085322,-0.0915406112613293,-0.0870190514838729,
-0.0784197287877601,-0.0545085386658457,-0.0392329067084975,-0.0154317870320417,
0.),.UNSPECIFIED.);
#351=B_SPLINE_CURVE_WITH_KNOTS('',3,(#12373,#12374,#12375,#12376,#12377,
#12378),.UNSPECIFIED.,.F.,.F.,(4,2,4),(-0.606706256981509,-0.303636876939173,
-0.00026974181288697),.UNSPECIFIED.);
#352=B_SPLINE_CURVE_WITH_KNOTS('',3,(#12396,#12397,#12398,#12399),
 .UNSPECIFIED.,.F.,.F.,(4,4),(0.0112334529114386,0.618489359031386),
 .UNSPECIFIED.);
#353=B_SPLINE_CURVE_WITH_KNOTS('',3,(#12400,#12401,#12402,#12403),
 .UNSPECIFIED.,.F.,.F.,(4,4),(-10.4271318523291,-9.85085636625011),
 .UNSPECIFIED.);
#354=B_SPLINE_CURVE_WITH_KNOTS('',3,(#12426,#12427,#12428,#12429),
 .UNSPECIFIED.,.F.,.F.,(4,4),(9.85750350611301,10.4271318523291),
 .UNSPECIFIED.);
#355=B_SPLINE_CURVE_WITH_KNOTS('',3,(#12433,#12434,#12435,#12436),
 .UNSPECIFIED.,.F.,.F.,(4,4),(0.27539863731415,0.845026983530265),
 .UNSPECIFIED.);
#356=B_SPLINE_CURVE_WITH_KNOTS('',3,(#12454,#12455,#12456,#12457),
 .UNSPECIFIED.,.F.,.F.,(4,4),(-0.851674123393175,-0.27539863731415),
 .UNSPECIFIED.);
#357=B_SPLINE_CURVE_WITH_KNOTS('',3,(#12458,#12459,#12460,#12461),
 .UNSPECIFIED.,.F.,.F.,(4,4),(-0.618489359031386,-0.0112334529114389),
 .UNSPECIFIED.);
#358=B_SPLINE_CURVE_WITH_KNOTS('',3,(#12541,#12542,#12543,#12544),
 .UNSPECIFIED.,.F.,.F.,(4,4),(0.0112755522169305,0.618164468641375),
 .UNSPECIFIED.);
#359=B_SPLINE_CURVE_WITH_KNOTS('',3,(#12565,#12566,#12567,#12568),
 .UNSPECIFIED.,.F.,.F.,(4,4),(-0.618164468641375,-0.0112755522169305),
 .UNSPECIFIED.);
#360=B_SPLINE_CURVE_WITH_KNOTS('',3,(#12654,#12655,#12656,#12657),
 .UNSPECIFIED.,.F.,.F.,(4,4),(5.55111512312578E-17,0.618489359031386),
 .UNSPECIFIED.);
#361=B_SPLINE_CURVE_WITH_KNOTS('',3,(#12658,#12659,#12660,#12661),
 .UNSPECIFIED.,.F.,.F.,(4,4),(-0.618489359031386,-0.00110654915602034),
 .UNSPECIFIED.);
#362=B_SPLINE_CURVE_WITH_KNOTS('',3,(#12697,#12698,#12699,#12700,#12701),
 .UNSPECIFIED.,.F.,.F.,(4,1,4),(-10.4271318523291,-4.63063308449434,-0.283259008618247),
 .UNSPECIFIED.);
#363=B_SPLINE_CURVE_WITH_KNOTS('',3,(#12702,#12703,#12704,#12705,#12706),
 .UNSPECIFIED.,.F.,.F.,(4,1,4),(0.283259011433087,4.63063308449434,10.4271318523291),
 .UNSPECIFIED.);
#364=B_SPLINE_CURVE_WITH_KNOTS('',3,(#12727,#12728,#12729,#12730),
 .UNSPECIFIED.,.F.,.F.,(4,4),(0.000779732613545348,0.618164468641375),
 .UNSPECIFIED.);
#365=B_SPLINE_CURVE_WITH_KNOTS('',3,(#12731,#12732,#12733,#12734),
 .UNSPECIFIED.,.F.,.F.,(4,4),(-0.618164468641375,-4.9439619065339E-17),
 .UNSPECIFIED.);
#366=B_SPLINE_CURVE_WITH_KNOTS('',3,(#12755,#12756,#12757,#12758),
 .UNSPECIFIED.,.F.,.F.,(4,4),(3.0964814046186E-16,0.618164468641375),
 .UNSPECIFIED.);
#367=B_SPLINE_CURVE_WITH_KNOTS('',3,(#12759,#12760,#12761,#12762),
 .UNSPECIFIED.,.F.,.F.,(4,4),(-0.618164468641375,-0.0007797326135453),
 .UNSPECIFIED.);
#368=B_SPLINE_CURVE_WITH_KNOTS('',3,(#12788,#12789,#12790,#12791,#12792),
 .UNSPECIFIED.,.F.,.F.,(4,1,4),(-10.419271481025,-4.62277271319024,-0.27539863731415),
 .UNSPECIFIED.);
#369=B_SPLINE_CURVE_WITH_KNOTS('',3,(#12793,#12794,#12795,#12796,#12797),
 .UNSPECIFIED.,.F.,.F.,(4,1,4),(0.27539863731415,4.62277271319024,10.419271481025),
 .UNSPECIFIED.);
#370=B_SPLINE_CURVE_WITH_KNOTS('',3,(#12818,#12819,#12820,#12821),
 .UNSPECIFIED.,.F.,.F.,(4,4),(0.00110654915602046,0.618489359031386),
 .UNSPECIFIED.);
#371=B_SPLINE_CURVE_WITH_KNOTS('',3,(#12822,#12823,#12824,#12825),
 .UNSPECIFIED.,.F.,.F.,(4,4),(-0.618489359031386,6.93889390390723E-18),
 .UNSPECIFIED.);
#558=SHAPE_REPRESENTATION_RELATIONSHIP('SRR','None',#18629,#567);
#567=ADVANCED_BREP_SHAPE_REPRESENTATION('',(#585),#18575);
#576=STYLED_ITEM('',(#18686),#585);
#585=MANIFOLD_SOLID_BREP('Body1',#6548);
#616=FACE_BOUND('',#1340,.T.);
#617=FACE_BOUND('',#1341,.T.);
#618=FACE_BOUND('',#1342,.T.);
#619=FACE_BOUND('',#1350,.T.);
#620=FACE_BOUND('',#1358,.T.);
#621=FACE_BOUND('',#1373,.T.);
#622=FACE_BOUND('',#1375,.T.);
#623=FACE_BOUND('',#1387,.T.);
#624=FACE_BOUND('',#1408,.T.);
#625=FACE_BOUND('',#1409,.T.);
#626=FACE_BOUND('',#1410,.T.);
#627=FACE_BOUND('',#1445,.T.);
#628=FACE_BOUND('',#1446,.T.);
#629=FACE_BOUND('',#1447,.T.);
#630=FACE_BOUND('',#1448,.T.);
#631=FACE_BOUND('',#1449,.T.);
#632=FACE_BOUND('',#1450,.T.);
#717=PLANE('',#6841);
#718=PLANE('',#6845);
#719=PLANE('',#6846);
#720=PLANE('',#6847);
#721=PLANE('',#6848);
#722=PLANE('',#6849);
#723=PLANE('',#6850);
#724=PLANE('',#6851);
#725=PLANE('',#6853);
#726=PLANE('',#6854);
#727=PLANE('',#6855);
#728=PLANE('',#6856);
#729=PLANE('',#6857);
#730=PLANE('',#6858);
#731=PLANE('',#6859);
#732=PLANE('',#6875);
#733=PLANE('',#6876);
#734=PLANE('',#6877);
#735=PLANE('',#6878);
#736=PLANE('',#6879);
#737=PLANE('',#6880);
#738=PLANE('',#6881);
#739=PLANE('',#6882);
#740=PLANE('',#6884);
#741=PLANE('',#6886);
#742=PLANE('',#6887);
#743=PLANE('',#6888);
#744=PLANE('',#6889);
#745=PLANE('',#6890);
#746=PLANE('',#6891);
#747=PLANE('',#6892);
#748=PLANE('',#6893);
#749=PLANE('',#6894);
#750=PLANE('',#6895);
#751=PLANE('',#6896);
#752=PLANE('',#6900);
#753=PLANE('',#6902);
#754=PLANE('',#6903);
#755=PLANE('',#6904);
#756=PLANE('',#6905);
#757=PLANE('',#6906);
#758=PLANE('',#6907);
#759=PLANE('',#6909);
#760=PLANE('',#6926);
#761=PLANE('',#6945);
#762=PLANE('',#6946);
#763=PLANE('',#6947);
#931=FACE_OUTER_BOUND('',#1333,.T.);
#932=FACE_OUTER_BOUND('',#1334,.T.);
#933=FACE_OUTER_BOUND('',#1335,.T.);
#934=FACE_OUTER_BOUND('',#1336,.T.);
#935=FACE_OUTER_BOUND('',#1337,.T.);
#936=FACE_OUTER_BOUND('',#1338,.T.);
#937=FACE_OUTER_BOUND('',#1339,.T.);
#938=FACE_OUTER_BOUND('',#1343,.T.);
#939=FACE_OUTER_BOUND('',#1344,.T.);
#940=FACE_OUTER_BOUND('',#1345,.T.);
#941=FACE_OUTER_BOUND('',#1346,.T.);
#942=FACE_OUTER_BOUND('',#1347,.T.);
#943=FACE_OUTER_BOUND('',#1348,.T.);
#944=FACE_OUTER_BOUND('',#1349,.T.);
#945=FACE_OUTER_BOUND('',#1351,.T.);
#946=FACE_OUTER_BOUND('',#1352,.T.);
#947=FACE_OUTER_BOUND('',#1353,.T.);
#948=FACE_OUTER_BOUND('',#1354,.T.);
#949=FACE_OUTER_BOUND('',#1355,.T.);
#950=FACE_OUTER_BOUND('',#1356,.T.);
#951=FACE_OUTER_BOUND('',#1357,.T.);
#952=FACE_OUTER_BOUND('',#1359,.T.);
#953=FACE_OUTER_BOUND('',#1360,.T.);
#954=FACE_OUTER_BOUND('',#1361,.T.);
#955=FACE_OUTER_BOUND('',#1362,.T.);
#956=FACE_OUTER_BOUND('',#1363,.T.);
#957=FACE_OUTER_BOUND('',#1364,.T.);
#958=FACE_OUTER_BOUND('',#1365,.T.);
#959=FACE_OUTER_BOUND('',#1366,.T.);
#960=FACE_OUTER_BOUND('',#1367,.T.);
#961=FACE_OUTER_BOUND('',#1368,.T.);
#962=FACE_OUTER_BOUND('',#1369,.T.);
#963=FACE_OUTER_BOUND('',#1370,.T.);
#964=FACE_OUTER_BOUND('',#1371,.T.);
#965=FACE_OUTER_BOUND('',#1372,.T.);
#966=FACE_OUTER_BOUND('',#1374,.T.);
#967=FACE_OUTER_BOUND('',#1376,.T.);
#968=FACE_OUTER_BOUND('',#1377,.T.);
#969=FACE_OUTER_BOUND('',#1378,.T.);
#970=FACE_OUTER_BOUND('',#1379,.T.);
#971=FACE_OUTER_BOUND('',#1380,.T.);
#972=FACE_OUTER_BOUND('',#1381,.T.);
#973=FACE_OUTER_BOUND('',#1382,.T.);
#974=FACE_OUTER_BOUND('',#1383,.T.);
#975=FACE_OUTER_BOUND('',#1384,.T.);
#976=FACE_OUTER_BOUND('',#1385,.T.);
#977=FACE_OUTER_BOUND('',#1386,.T.);
#978=FACE_OUTER_BOUND('',#1388,.T.);
#979=FACE_OUTER_BOUND('',#1389,.T.);
#980=FACE_OUTER_BOUND('',#1390,.T.);
#981=FACE_OUTER_BOUND('',#1391,.T.);
#982=FACE_OUTER_BOUND('',#1392,.T.);
#983=FACE_OUTER_BOUND('',#1393,.T.);
#984=FACE_OUTER_BOUND('',#1394,.T.);
#985=FACE_OUTER_BOUND('',#1395,.T.);
#986=FACE_OUTER_BOUND('',#1396,.T.);
#987=FACE_OUTER_BOUND('',#1397,.T.);
#988=FACE_OUTER_BOUND('',#1398,.T.);
#989=FACE_OUTER_BOUND('',#1399,.T.);
#990=FACE_OUTER_BOUND('',#1400,.T.);
#991=FACE_OUTER_BOUND('',#1401,.T.);
#992=FACE_OUTER_BOUND('',#1402,.T.);
#993=FACE_OUTER_BOUND('',#1403,.T.);
#994=FACE_OUTER_BOUND('',#1404,.T.);
#995=FACE_OUTER_BOUND('',#1405,.T.);
#996=FACE_OUTER_BOUND('',#1406,.T.);
#997=FACE_OUTER_BOUND('',#1407,.T.);
#998=FACE_OUTER_BOUND('',#1411,.T.);
#999=FACE_OUTER_BOUND('',#1412,.T.);
#1000=FACE_OUTER_BOUND('',#1413,.T.);
#1001=FACE_OUTER_BOUND('',#1414,.T.);
#1002=FACE_OUTER_BOUND('',#1415,.T.);
#1003=FACE_OUTER_BOUND('',#1416,.T.);
#1004=FACE_OUTER_BOUND('',#1417,.T.);
#1005=FACE_OUTER_BOUND('',#1418,.T.);
#1006=FACE_OUTER_BOUND('',#1419,.T.);
#1007=FACE_OUTER_BOUND('',#1420,.T.);
#1008=FACE_OUTER_BOUND('',#1421,.T.);
#1009=FACE_OUTER_BOUND('',#1422,.T.);
#1010=FACE_OUTER_BOUND('',#1423,.T.);
#1011=FACE_OUTER_BOUND('',#1424,.T.);
#1012=FACE_OUTER_BOUND('',#1425,.T.);
#1013=FACE_OUTER_BOUND('',#1426,.T.);
#1014=FACE_OUTER_BOUND('',#1427,.T.);
#1015=FACE_OUTER_BOUND('',#1428,.T.);
#1016=FACE_OUTER_BOUND('',#1429,.T.);
#1017=FACE_OUTER_BOUND('',#1430,.T.);
#1018=FACE_OUTER_BOUND('',#1431,.T.);
#1019=FACE_OUTER_BOUND('',#1432,.T.);
#1020=FACE_OUTER_BOUND('',#1433,.T.);
#1021=FACE_OUTER_BOUND('',#1434,.T.);
#1022=FACE_OUTER_BOUND('',#1435,.T.);
#1023=FACE_OUTER_BOUND('',#1436,.T.);
#1024=FACE_OUTER_BOUND('',#1437,.T.);
#1025=FACE_OUTER_BOUND('',#1438,.T.);
#1026=FACE_OUTER_BOUND('',#1439,.T.);
#1027=FACE_OUTER_BOUND('',#1440,.T.);
#1028=FACE_OUTER_BOUND('',#1441,.T.);
#1029=FACE_OUTER_BOUND('',#1442,.T.);
#1030=FACE_OUTER_BOUND('',#1443,.T.);
#1031=FACE_OUTER_BOUND('',#1444,.T.);
#1032=FACE_OUTER_BOUND('',#1451,.T.);
#1033=FACE_OUTER_BOUND('',#1452,.T.);
#1333=EDGE_LOOP('',(#4802,#4803));
#1334=EDGE_LOOP('',(#4804,#4805));
#1335=EDGE_LOOP('',(#4806,#4807));
#1336=EDGE_LOOP('',(#4808,#4809));
#1337=EDGE_LOOP('',(#4810,#4811,#4812,#4813,#4814,#4815));
#1338=EDGE_LOOP('',(#4816,#4817,#4818,#4819,#4820,#4821));
#1339=EDGE_LOOP('',(#4822,#4823,#4824,#4825,#4826,#4827,#4828,#4829));
#1340=EDGE_LOOP('',(#4830));
#1341=EDGE_LOOP('',(#4831));
#1342=EDGE_LOOP('',(#4832));
#1343=EDGE_LOOP('',(#4833,#4834,#4835,#4836));
#1344=EDGE_LOOP('',(#4837,#4838,#4839,#4840));
#1345=EDGE_LOOP('',(#4841,#4842,#4843,#4844));
#1346=EDGE_LOOP('',(#4845,#4846,#4847,#4848));
#1347=EDGE_LOOP('',(#4849,#4850,#4851,#4852));
#1348=EDGE_LOOP('',(#4853,#4854,#4855,#4856));
#1349=EDGE_LOOP('',(#4857,#4858,#4859,#4860,#4861,#4862));
#1350=EDGE_LOOP('',(#4863));
#1351=EDGE_LOOP('',(#4864,#4865,#4866,#4867));
#1352=EDGE_LOOP('',(#4868,#4869,#4870,#4871));
#1353=EDGE_LOOP('',(#4872,#4873,#4874,#4875));
#1354=EDGE_LOOP('',(#4876,#4877,#4878,#4879));
#1355=EDGE_LOOP('',(#4880,#4881,#4882,#4883));
#1356=EDGE_LOOP('',(#4884,#4885,#4886,#4887));
#1357=EDGE_LOOP('',(#4888,#4889,#4890,#4891,#4892,#4893));
#1358=EDGE_LOOP('',(#4894));
#1359=EDGE_LOOP('',(#4895,#4896,#4897,#4898));
#1360=EDGE_LOOP('',(#4899,#4900,#4901,#4902));
#1361=EDGE_LOOP('',(#4903,#4904,#4905,#4906));
#1362=EDGE_LOOP('',(#4907,#4908,#4909,#4910));
#1363=EDGE_LOOP('',(#4911,#4912,#4913,#4914));
#1364=EDGE_LOOP('',(#4915,#4916,#4917,#4918));
#1365=EDGE_LOOP('',(#4919,#4920,#4921,#4922));
#1366=EDGE_LOOP('',(#4923,#4924,#4925,#4926));
#1367=EDGE_LOOP('',(#4927,#4928,#4929,#4930));
#1368=EDGE_LOOP('',(#4931,#4932,#4933,#4934));
#1369=EDGE_LOOP('',(#4935,#4936,#4937,#4938));
#1370=EDGE_LOOP('',(#4939,#4940,#4941,#4942));
#1371=EDGE_LOOP('',(#4943,#4944,#4945,#4946));
#1372=EDGE_LOOP('',(#4947));
#1373=EDGE_LOOP('',(#4948));
#1374=EDGE_LOOP('',(#4949));
#1375=EDGE_LOOP('',(#4950));
#1376=EDGE_LOOP('',(#4951,#4952,#4953,#4954));
#1377=EDGE_LOOP('',(#4955,#4956,#4957,#4958));
#1378=EDGE_LOOP('',(#4959,#4960,#4961,#4962));
#1379=EDGE_LOOP('',(#4963,#4964,#4965,#4966));
#1380=EDGE_LOOP('',(#4967,#4968,#4969,#4970));
#1381=EDGE_LOOP('',(#4971,#4972,#4973,#4974,#4975,#4976));
#1382=EDGE_LOOP('',(#4977,#4978,#4979,#4980,#4981,#4982,#4983,#4984,#4985,
#4986));
#1383=EDGE_LOOP('',(#4987,#4988,#4989,#4990,#4991,#4992,#4993,#4994,#4995,
#4996));
#1384=EDGE_LOOP('',(#4997,#4998,#4999,#5000,#5001,#5002,#5003,#5004,#5005,
#5006));
#1385=EDGE_LOOP('',(#5007,#5008,#5009,#5010,#5011,#5012,#5013,#5014));
#1386=EDGE_LOOP('',(#5015,#5016,#5017,#5018,#5019,#5020,#5021,#5022,#5023,
#5024,#5025,#5026,#5027,#5028,#5029,#5030,#5031,#5032,#5033,#5034,#5035,
#5036,#5037,#5038,#5039,#5040,#5041,#5042,#5043,#5044,#5045,#5046,#5047,
#5048,#5049,#5050,#5051,#5052,#5053,#5054,#5055,#5056));
#1387=EDGE_LOOP('',(#5057,#5058,#5059,#5060,#5061,#5062));
#1388=EDGE_LOOP('',(#5063,#5064,#5065,#5066));
#1389=EDGE_LOOP('',(#5067,#5068,#5069,#5070));
#1390=EDGE_LOOP('',(#5071,#5072,#5073,#5074,#5075,#5076));
#1391=EDGE_LOOP('',(#5077,#5078,#5079,#5080));
#1392=EDGE_LOOP('',(#5081,#5082,#5083,#5084));
#1393=EDGE_LOOP('',(#5085,#5086,#5087,#5088,#5089,#5090));
#1394=EDGE_LOOP('',(#5091,#5092,#5093,#5094));
#1395=EDGE_LOOP('',(#5095,#5096,#5097,#5098));
#1396=EDGE_LOOP('',(#5099,#5100,#5101,#5102));
#1397=EDGE_LOOP('',(#5103,#5104,#5105,#5106));
#1398=EDGE_LOOP('',(#5107,#5108,#5109,#5110,#5111,#5112,#5113,#5114,#5115,
#5116));
#1399=EDGE_LOOP('',(#5117,#5118,#5119,#5120));
#1400=EDGE_LOOP('',(#5121,#5122,#5123,#5124));
#1401=EDGE_LOOP('',(#5125,#5126,#5127,#5128));
#1402=EDGE_LOOP('',(#5129,#5130,#5131,#5132));
#1403=EDGE_LOOP('',(#5133,#5134,#5135,#5136));
#1404=EDGE_LOOP('',(#5137,#5138,#5139,#5140,#5141,#5142,#5143,#5144,#5145,
#5146));
#1405=EDGE_LOOP('',(#5147,#5148,#5149,#5150));
#1406=EDGE_LOOP('',(#5151,#5152,#5153,#5154,#5155,#5156));
#1407=EDGE_LOOP('',(#5157,#5158,#5159,#5160,#5161,#5162,#5163,#5164));
#1408=EDGE_LOOP('',(#5165));
#1409=EDGE_LOOP('',(#5166));
#1410=EDGE_LOOP('',(#5167));
#1411=EDGE_LOOP('',(#5168,#5169,#5170,#5171));
#1412=EDGE_LOOP('',(#5172,#5173,#5174,#5175,#5176,#5177,#5178,#5179,#5180,
#5181));
#1413=EDGE_LOOP('',(#5182,#5183,#5184,#5185));
#1414=EDGE_LOOP('',(#5186,#5187,#5188,#5189));
#1415=EDGE_LOOP('',(#5190,#5191,#5192,#5193));
#1416=EDGE_LOOP('',(#5194,#5195,#5196,#5197));
#1417=EDGE_LOOP('',(#5198,#5199,#5200,#5201));
#1418=EDGE_LOOP('',(#5202,#5203,#5204));
#1419=EDGE_LOOP('',(#5205,#5206,#5207));
#1420=EDGE_LOOP('',(#5208,#5209,#5210));
#1421=EDGE_LOOP('',(#5211,#5212,#5213,#5214));
#1422=EDGE_LOOP('',(#5215,#5216,#5217,#5218));
#1423=EDGE_LOOP('',(#5219,#5220,#5221));
#1424=EDGE_LOOP('',(#5222,#5223,#5224,#5225));
#1425=EDGE_LOOP('',(#5226,#5227,#5228,#5229));
#1426=EDGE_LOOP('',(#5230,#5231,#5232,#5233));
#1427=EDGE_LOOP('',(#5234,#5235,#5236,#5237));
#1428=EDGE_LOOP('',(#5238,#5239,#5240,#5241));
#1429=EDGE_LOOP('',(#5242,#5243,#5244,#5245));
#1430=EDGE_LOOP('',(#5246,#5247,#5248));
#1431=EDGE_LOOP('',(#5249,#5250,#5251));
#1432=EDGE_LOOP('',(#5252,#5253,#5254));
#1433=EDGE_LOOP('',(#5255,#5256,#5257,#5258));
#1434=EDGE_LOOP('',(#5259,#5260,#5261,#5262));
#1435=EDGE_LOOP('',(#5263,#5264,#5265));
#1436=EDGE_LOOP('',(#5266,#5267,#5268,#5269));
#1437=EDGE_LOOP('',(#5270,#5271,#5272,#5273));
#1438=EDGE_LOOP('',(#5274,#5275,#5276,#5277));
#1439=EDGE_LOOP('',(#5278,#5279,#5280,#5281));
#1440=EDGE_LOOP('',(#5282,#5283,#5284,#5285));
#1441=EDGE_LOOP('',(#5286,#5287,#5288,#5289));
#1442=EDGE_LOOP('',(#5290,#5291,#5292,#5293));
#1443=EDGE_LOOP('',(#5294,#5295,#5296,#5297,#5298,#5299,#5300,#5301));
#1444=EDGE_LOOP('',(#5302,#5303,#5304,#5305));
#1445=EDGE_LOOP('',(#5306,#5307,#5308,#5309,#5310,#5311));
#1446=EDGE_LOOP('',(#5312,#5313,#5314,#5315,#5316,#5317));
#1447=EDGE_LOOP('',(#5318));
#1448=EDGE_LOOP('',(#5319));
#1449=EDGE_LOOP('',(#5320));
#1450=EDGE_LOOP('',(#5321));
#1451=EDGE_LOOP('',(#5322,#5323,#5324,#5325));
#1452=EDGE_LOOP('',(#5326,#5327,#5328,#5329));
#1770=LINE('',#11051,#2177);
#1771=LINE('',#11053,#2178);
#1772=LINE('',#11067,#2179);
#1773=LINE('',#11069,#2180);
#1774=LINE('',#11071,#2181);
#1775=LINE('',#11072,#2182);
#1776=LINE('',#11075,#2183);
#1777=LINE('',#11077,#2184);
#1778=LINE('',#11078,#2185);
#1779=LINE('',#11081,#2186);
#1780=LINE('',#11083,#2187);
#1781=LINE('',#11084,#2188);
#1782=LINE('',#11087,#2189);
#1783=LINE('',#11089,#2190);
#1784=LINE('',#11090,#2191);
#1785=LINE('',#11093,#2192);
#1786=LINE('',#11095,#2193);
#1787=LINE('',#11096,#2194);
#1788=LINE('',#11098,#2195);
#1789=LINE('',#11099,#2196);
#1790=LINE('',#11106,#2197);
#1791=LINE('',#11108,#2198);
#1792=LINE('',#11110,#2199);
#1793=LINE('',#11111,#2200);
#1794=LINE('',#11114,#2201);
#1795=LINE('',#11116,#2202);
#1796=LINE('',#11117,#2203);
#1797=LINE('',#11120,#2204);
#1798=LINE('',#11122,#2205);
#1799=LINE('',#11123,#2206);
#1800=LINE('',#11126,#2207);
#1801=LINE('',#11128,#2208);
#1802=LINE('',#11129,#2209);
#1803=LINE('',#11132,#2210);
#1804=LINE('',#11134,#2211);
#1805=LINE('',#11135,#2212);
#1806=LINE('',#11137,#2213);
#1807=LINE('',#11138,#2214);
#1808=LINE('',#11145,#2215);
#1809=LINE('',#11150,#2216);
#1810=LINE('',#11156,#2217);
#1811=LINE('',#11161,#2218);
#1812=LINE('',#11164,#2219);
#1813=LINE('',#11168,#2220);
#1814=LINE('',#11173,#2221);
#1815=LINE('',#11175,#2222);
#1816=LINE('',#11177,#2223);
#1817=LINE('',#11178,#2224);
#1818=LINE('',#11182,#2225);
#1819=LINE('',#11184,#2226);
#1820=LINE('',#11186,#2227);
#1821=LINE('',#11187,#2228);
#1822=LINE('',#11191,#2229);
#1823=LINE('',#11193,#2230);
#1824=LINE('',#11195,#2231);
#1825=LINE('',#11196,#2232);
#1826=LINE('',#11200,#2233);
#1827=LINE('',#11202,#2234);
#1828=LINE('',#11204,#2235);
#1829=LINE('',#11205,#2236);
#1830=LINE('',#11209,#2237);
#1831=LINE('',#11211,#2238);
#1832=LINE('',#11213,#2239);
#1833=LINE('',#11214,#2240);
#1834=LINE('',#11218,#2241);
#1835=LINE('',#11220,#2242);
#1836=LINE('',#11222,#2243);
#1837=LINE('',#11223,#2244);
#1838=LINE('',#11227,#2245);
#1839=LINE('',#11229,#2246);
#1840=LINE('',#11231,#2247);
#1841=LINE('',#11232,#2248);
#1842=LINE('',#11240,#2249);
#1843=LINE('',#11241,#2250);
#1844=LINE('',#11243,#2251);
#1845=LINE('',#11244,#2252);
#1846=LINE('',#11246,#2253);
#1847=LINE('',#11247,#2254);
#1848=LINE('',#11250,#2255);
#1849=LINE('',#11252,#2256);
#1850=LINE('',#11253,#2257);
#1851=LINE('',#11256,#2258);
#1852=LINE('',#11258,#2259);
#1853=LINE('',#11259,#2260);
#1854=LINE('',#11263,#2261);
#1855=LINE('',#11307,#2262);
#1856=LINE('',#11350,#2263);
#1857=LINE('',#11353,#2264);
#1858=LINE('',#11391,#2265);
#1859=LINE('',#11428,#2266);
#1860=LINE('',#11431,#2267);
#1861=LINE('',#11439,#2268);
#1862=LINE('',#11476,#2269);
#1863=LINE('',#11479,#2270);
#1864=LINE('',#11486,#2271);
#1865=LINE('',#11492,#2272);
#1866=LINE('',#11503,#2273);
#1867=LINE('',#11512,#2274);
#1868=LINE('',#11518,#2275);
#1869=LINE('',#11553,#2276);
#1870=LINE('',#11624,#2277);
#1871=LINE('',#11694,#2278);
#1872=LINE('',#11726,#2279);
#1873=LINE('',#11732,#2280);
#1874=LINE('',#11741,#2281);
#1875=LINE('',#11778,#2282);
#1876=LINE('',#11813,#2283);
#1877=LINE('',#11815,#2284);
#1878=LINE('',#11819,#2285);
#1879=LINE('',#11865,#2286);
#1880=LINE('',#11991,#2287);
#1881=LINE('',#12071,#2288);
#1882=LINE('',#12233,#2289);
#1883=LINE('',#12343,#2290);
#1884=LINE('',#12432,#2291);
#1885=LINE('',#12520,#2292);
#1886=LINE('',#12632,#2293);
#1887=LINE('',#12633,#2294);
#1888=LINE('',#12670,#2295);
#1889=LINE('',#12671,#2296);
#2177=VECTOR('',#7673,1.);
#2178=VECTOR('',#7674,1.);
#2179=VECTOR('',#7683,1.);
#2180=VECTOR('',#7684,1.);
#2181=VECTOR('',#7685,1.);
#2182=VECTOR('',#7686,1.);
#2183=VECTOR('',#7689,1.);
#2184=VECTOR('',#7690,1.);
#2185=VECTOR('',#7691,1.);
#2186=VECTOR('',#7694,1.);
#2187=VECTOR('',#7695,1.);
#2188=VECTOR('',#7696,1.);
#2189=VECTOR('',#7699,1.);
#2190=VECTOR('',#7700,1.);
#2191=VECTOR('',#7701,1.);
#2192=VECTOR('',#7704,1.);
#2193=VECTOR('',#7705,1.);
#2194=VECTOR('',#7706,1.);
#2195=VECTOR('',#7709,1.);
#2196=VECTOR('',#7710,1.);
#2197=VECTOR('',#7717,1.);
#2198=VECTOR('',#7718,1.);
#2199=VECTOR('',#7719,1.);
#2200=VECTOR('',#7720,1.);
#2201=VECTOR('',#7723,1.);
#2202=VECTOR('',#7724,1.);
#2203=VECTOR('',#7725,1.);
#2204=VECTOR('',#7728,1.);
#2205=VECTOR('',#7729,1.);
#2206=VECTOR('',#7730,1.);
#2207=VECTOR('',#7733,1.);
#2208=VECTOR('',#7734,1.);
#2209=VECTOR('',#7735,1.);
#2210=VECTOR('',#7738,1.);
#2211=VECTOR('',#7739,1.);
#2212=VECTOR('',#7740,1.);
#2213=VECTOR('',#7743,1.);
#2214=VECTOR('',#7744,1.);
#2215=VECTOR('',#7753,0.15);
#2216=VECTOR('',#7758,0.15);
#2217=VECTOR('',#7765,0.15);
#2218=VECTOR('',#7772,0.15);
#2219=VECTOR('',#7775,0.17);
#2220=VECTOR('',#7780,0.17);
#2221=VECTOR('',#7785,1.);
#2222=VECTOR('',#7786,1.);
#2223=VECTOR('',#7787,1.);
#2224=VECTOR('',#7788,1.);
#2225=VECTOR('',#7791,1.);
#2226=VECTOR('',#7792,1.);
#2227=VECTOR('',#7793,1.);
#2228=VECTOR('',#7794,1.);
#2229=VECTOR('',#7797,1.);
#2230=VECTOR('',#7798,1.);
#2231=VECTOR('',#7799,1.);
#2232=VECTOR('',#7800,1.);
#2233=VECTOR('',#7803,1.);
#2234=VECTOR('',#7804,1.);
#2235=VECTOR('',#7805,1.);
#2236=VECTOR('',#7806,1.);
#2237=VECTOR('',#7809,1.);
#2238=VECTOR('',#7810,1.);
#2239=VECTOR('',#7811,1.);
#2240=VECTOR('',#7812,1.);
#2241=VECTOR('',#7815,1.);
#2242=VECTOR('',#7816,1.);
#2243=VECTOR('',#7817,1.);
#2244=VECTOR('',#7818,1.);
#2245=VECTOR('',#7821,1.);
#2246=VECTOR('',#7822,1.);
#2247=VECTOR('',#7823,1.);
#2248=VECTOR('',#7824,1.);
#2249=VECTOR('',#7835,1.);
#2250=VECTOR('',#7836,1.);
#2251=VECTOR('',#7839,1.);
#2252=VECTOR('',#7840,1.);
#2253=VECTOR('',#7843,1.);
#2254=VECTOR('',#7844,1.);
#2255=VECTOR('',#7847,1.);
#2256=VECTOR('',#7848,1.);
#2257=VECTOR('',#7849,1.);
#2258=VECTOR('',#7852,1.);
#2259=VECTOR('',#7853,1.);
#2260=VECTOR('',#7854,1.);
#2261=VECTOR('',#7857,1.);
#2262=VECTOR('',#7860,1.);
#2263=VECTOR('',#7861,1.);
#2264=VECTOR('',#7864,1.);
#2265=VECTOR('',#7865,1.);
#2266=VECTOR('',#7866,1.);
#2267=VECTOR('',#7869,1.);
#2268=VECTOR('',#7870,1.);
#2269=VECTOR('',#7871,1.);
#2270=VECTOR('',#7874,1.);
#2271=VECTOR('',#7875,1.);
#2272=VECTOR('',#7876,1.);
#2273=VECTOR('',#7879,1.);
#2274=VECTOR('',#7880,1.);
#2275=VECTOR('',#7881,1.);
#2276=VECTOR('',#7882,1.);
#2277=VECTOR('',#7883,1.);
#2278=VECTOR('',#7884,1.);
#2279=VECTOR('',#7885,1.);
#2280=VECTOR('',#7886,1.);
#2281=VECTOR('',#7887,1.);
#2282=VECTOR('',#7888,1.);
#2283=VECTOR('',#7889,1.);
#2284=VECTOR('',#7892,0.4);
#2285=VECTOR('',#7897,0.4);
#2286=VECTOR('',#7900,1.);
#2287=VECTOR('',#7905,1.);
#2288=VECTOR('',#7908,1.);
#2289=VECTOR('',#7913,1.);
#2290=VECTOR('',#7918,1.);
#2291=VECTOR('',#7923,1.);
#2292=VECTOR('',#7956,1.);
#2293=VECTOR('',#7985,1.);
#2294=VECTOR('',#7986,1.);
#2295=VECTOR('',#7997,1.);
#2296=VECTOR('',#7998,1.);
#2493=CIRCLE('',#6834,0.25);
#2494=CIRCLE('',#6836,0.25);
#2495=CIRCLE('',#6838,0.25);
#2496=CIRCLE('',#6840,0.25);
#2497=CIRCLE('',#6842,0.15);
#2498=CIRCLE('',#6843,0.15);
#2499=CIRCLE('',#6844,0.4);
#2500=CIRCLE('',#6852,0.17);
#2501=CIRCLE('',#6860,0.17);
#2502=CIRCLE('',#6862,0.15);
#2503=CIRCLE('',#6864,0.15);
#2504=CIRCLE('',#6865,0.15);
#2505=CIRCLE('',#6867,0.15);
#2506=CIRCLE('',#6868,0.15);
#2507=CIRCLE('',#6870,0.15);
#2508=CIRCLE('',#6872,0.17);
#2509=CIRCLE('',#6874,0.17);
#2510=CIRCLE('',#6883,0.4);
#2511=CIRCLE('',#6885,0.4);
#2512=CIRCLE('',#6899,0.4);
#2513=CIRCLE('',#6901,0.1);
#2514=CIRCLE('',#6908,0.0999999999999995);
#2515=CIRCLE('',#6910,0.1);
#2516=CIRCLE('',#6912,0.1);
#2517=CIRCLE('',#6913,0.1);
#2518=CIRCLE('',#6915,0.0999999999999999);
#2519=CIRCLE('',#6916,0.0999999999999998);
#2520=CIRCLE('',#6917,0.0999999999999998);
#2521=CIRCLE('',#6919,0.0999999999999994);
#2522=CIRCLE('',#6920,0.0999999999999993);
#2523=CIRCLE('',#6923,0.0999999999999999);
#2524=CIRCLE('',#6924,0.1);
#2525=CIRCLE('',#6928,0.3);
#2526=CIRCLE('',#6929,0.3);
#2527=CIRCLE('',#6930,0.3);
#2528=CIRCLE('',#6932,0.3);
#2529=CIRCLE('',#6933,0.3);
#2530=CIRCLE('',#6934,0.3);
#2531=CIRCLE('',#6936,0.3);
#2532=CIRCLE('',#6937,0.299999999999999);
#2533=CIRCLE('',#6938,0.3);
#2534=CIRCLE('',#6941,0.3);
#2535=CIRCLE('',#6942,0.3);
#2536=CIRCLE('',#6943,0.3);
#2793=VERTEX_POINT('',#10758);
#2794=VERTEX_POINT('',#10759);
#2795=VERTEX_POINT('',#10786);
#2796=VERTEX_POINT('',#10787);
#2797=VERTEX_POINT('',#10810);
#2798=VERTEX_POINT('',#10811);
#2799=VERTEX_POINT('',#10834);
#2800=VERTEX_POINT('',#10835);
#2801=VERTEX_POINT('',#10881);
#2802=VERTEX_POINT('',#10886);
#2803=VERTEX_POINT('',#10915);
#2804=VERTEX_POINT('',#10920);
#2805=VERTEX_POINT('',#10973);
#2806=VERTEX_POINT('',#10978);
#2807=VERTEX_POINT('',#11007);
#2808=VERTEX_POINT('',#11012);
#2809=VERTEX_POINT('',#11046);
#2810=VERTEX_POINT('',#11052);
#2811=VERTEX_POINT('',#11058);
#2812=VERTEX_POINT('',#11060);
#2813=VERTEX_POINT('',#11062);
#2814=VERTEX_POINT('',#11065);
#2815=VERTEX_POINT('',#11066);
#2816=VERTEX_POINT('',#11068);
#2817=VERTEX_POINT('',#11070);
#2818=VERTEX_POINT('',#11074);
#2819=VERTEX_POINT('',#11076);
#2820=VERTEX_POINT('',#11080);
#2821=VERTEX_POINT('',#11082);
#2822=VERTEX_POINT('',#11086);
#2823=VERTEX_POINT('',#11088);
#2824=VERTEX_POINT('',#11092);
#2825=VERTEX_POINT('',#11094);
#2826=VERTEX_POINT('',#11101);
#2827=VERTEX_POINT('',#11104);
#2828=VERTEX_POINT('',#11105);
#2829=VERTEX_POINT('',#11107);
#2830=VERTEX_POINT('',#11109);
#2831=VERTEX_POINT('',#11113);
#2832=VERTEX_POINT('',#11115);
#2833=VERTEX_POINT('',#11119);
#2834=VERTEX_POINT('',#11121);
#2835=VERTEX_POINT('',#11125);
#2836=VERTEX_POINT('',#11127);
#2837=VERTEX_POINT('',#11131);
#2838=VERTEX_POINT('',#11133);
#2839=VERTEX_POINT('',#11140);
#2840=VERTEX_POINT('',#11143);
#2841=VERTEX_POINT('',#11147);
#2842=VERTEX_POINT('',#11149);
#2843=VERTEX_POINT('',#11153);
#2844=VERTEX_POINT('',#11155);
#2845=VERTEX_POINT('',#11159);
#2846=VERTEX_POINT('',#11163);
#2847=VERTEX_POINT('',#11167);
#2848=VERTEX_POINT('',#11171);
#2849=VERTEX_POINT('',#11172);
#2850=VERTEX_POINT('',#11174);
#2851=VERTEX_POINT('',#11176);
#2852=VERTEX_POINT('',#11180);
#2853=VERTEX_POINT('',#11181);
#2854=VERTEX_POINT('',#11183);
#2855=VERTEX_POINT('',#11185);
#2856=VERTEX_POINT('',#11189);
#2857=VERTEX_POINT('',#11190);
#2858=VERTEX_POINT('',#11192);
#2859=VERTEX_POINT('',#11194);
#2860=VERTEX_POINT('',#11198);
#2861=VERTEX_POINT('',#11199);
#2862=VERTEX_POINT('',#11201);
#2863=VERTEX_POINT('',#11203);
#2864=VERTEX_POINT('',#11207);
#2865=VERTEX_POINT('',#11208);
#2866=VERTEX_POINT('',#11210);
#2867=VERTEX_POINT('',#11212);
#2868=VERTEX_POINT('',#11216);
#2869=VERTEX_POINT('',#11217);
#2870=VERTEX_POINT('',#11219);
#2871=VERTEX_POINT('',#11221);
#2872=VERTEX_POINT('',#11225);
#2873=VERTEX_POINT('',#11226);
#2874=VERTEX_POINT('',#11228);
#2875=VERTEX_POINT('',#11230);
#2876=VERTEX_POINT('',#11234);
#2877=VERTEX_POINT('',#11237);
#2878=VERTEX_POINT('',#11249);
#2879=VERTEX_POINT('',#11251);
#2880=VERTEX_POINT('',#11255);
#2881=VERTEX_POINT('',#11257);
#2882=VERTEX_POINT('',#11261);
#2883=VERTEX_POINT('',#11262);
#2884=VERTEX_POINT('',#11264);
#2885=VERTEX_POINT('',#11306);
#2886=VERTEX_POINT('',#11314);
#2887=VERTEX_POINT('',#11343);
#2888=VERTEX_POINT('',#11352);
#2889=VERTEX_POINT('',#11354);
#2890=VERTEX_POINT('',#11361);
#2891=VERTEX_POINT('',#11390);
#2892=VERTEX_POINT('',#11392);
#2893=VERTEX_POINT('',#11421);
#2894=VERTEX_POINT('',#11430);
#2895=VERTEX_POINT('',#11438);
#2896=VERTEX_POINT('',#11440);
#2897=VERTEX_POINT('',#11469);
#2898=VERTEX_POINT('',#11478);
#2899=VERTEX_POINT('',#11480);
#2900=VERTEX_POINT('',#11485);
#2901=VERTEX_POINT('',#11487);
#2902=VERTEX_POINT('',#11502);
#2903=VERTEX_POINT('',#11511);
#2904=VERTEX_POINT('',#11517);
#2905=VERTEX_POINT('',#11519);
#2906=VERTEX_POINT('',#11552);
#2907=VERTEX_POINT('',#11554);
#2908=VERTEX_POINT('',#11586);
#2909=VERTEX_POINT('',#11591);
#2910=VERTEX_POINT('',#11623);
#2911=VERTEX_POINT('',#11625);
#2912=VERTEX_POINT('',#11657);
#2913=VERTEX_POINT('',#11662);
#2914=VERTEX_POINT('',#11695);
#2915=VERTEX_POINT('',#11721);
#2916=VERTEX_POINT('',#11727);
#2917=VERTEX_POINT('',#11733);
#2918=VERTEX_POINT('',#11742);
#2919=VERTEX_POINT('',#11743);
#2920=VERTEX_POINT('',#11748);
#2921=VERTEX_POINT('',#11777);
#2922=VERTEX_POINT('',#11779);
#2923=VERTEX_POINT('',#11808);
#2924=VERTEX_POINT('',#11817);
#2925=VERTEX_POINT('',#11821);
#2926=VERTEX_POINT('',#11828);
#2927=VERTEX_POINT('',#11835);
#2928=VERTEX_POINT('',#11864);
#2929=VERTEX_POINT('',#11930);
#2930=VERTEX_POINT('',#11979);
#2931=VERTEX_POINT('',#11986);
#2932=VERTEX_POINT('',#12024);
#2933=VERTEX_POINT('',#12034);
#2934=VERTEX_POINT('',#12041);
#2935=VERTEX_POINT('',#12070);
#2936=VERTEX_POINT('',#12072);
#2937=VERTEX_POINT('',#12197);
#2938=VERTEX_POINT('',#12204);
#2939=VERTEX_POINT('',#12306);
#2940=VERTEX_POINT('',#12313);
#2941=VERTEX_POINT('',#12342);
#2942=VERTEX_POINT('',#12344);
#2943=VERTEX_POINT('',#12395);
#2944=VERTEX_POINT('',#12424);
#2945=VERTEX_POINT('',#12431);
#2946=VERTEX_POINT('',#12453);
#2947=VERTEX_POINT('',#12488);
#2948=VERTEX_POINT('',#12516);
#2949=VERTEX_POINT('',#12611);
#2950=VERTEX_POINT('',#12612);
#2951=VERTEX_POINT('',#12614);
#2952=VERTEX_POINT('',#12618);
#2953=VERTEX_POINT('',#12619);
#2954=VERTEX_POINT('',#12621);
#2955=VERTEX_POINT('',#12625);
#2956=VERTEX_POINT('',#12626);
#2957=VERTEX_POINT('',#12628);
#2958=VERTEX_POINT('',#12663);
#2959=VERTEX_POINT('',#12664);
#2960=VERTEX_POINT('',#12666);
#3524=EDGE_CURVE('',#2793,#2794,#272,.T.);
#3525=EDGE_CURVE('',#2793,#2794,#2493,.T.);
#3526=EDGE_CURVE('',#2795,#2796,#273,.T.);
#3527=EDGE_CURVE('',#2795,#2796,#2494,.T.);
#3528=EDGE_CURVE('',#2797,#2798,#274,.T.);
#3529=EDGE_CURVE('',#2797,#2798,#2495,.T.);
#3530=EDGE_CURVE('',#2799,#2800,#275,.T.);
#3531=EDGE_CURVE('',#2799,#2800,#2496,.T.);
#3532=EDGE_CURVE('',#2801,#2796,#276,.T.);
#3533=EDGE_CURVE('',#2801,#2802,#277,.T.);
#3534=EDGE_CURVE('',#2803,#2802,#278,.T.);
#3535=EDGE_CURVE('',#2803,#2804,#279,.T.);
#3536=EDGE_CURVE('',#2795,#2804,#280,.T.);
#3537=EDGE_CURVE('',#2805,#2800,#281,.T.);
#3538=EDGE_CURVE('',#2805,#2806,#282,.T.);
#3539=EDGE_CURVE('',#2807,#2806,#283,.T.);
#3540=EDGE_CURVE('',#2807,#2808,#284,.T.);
#3541=EDGE_CURVE('',#2799,#2808,#285,.T.);
#3542=EDGE_CURVE('',#2793,#2809,#286,.T.);
#3543=EDGE_CURVE('',#2809,#2805,#1770,.T.);
#3544=EDGE_CURVE('',#2808,#2810,#1771,.T.);
#3545=EDGE_CURVE('',#2810,#2794,#287,.T.);
#3546=EDGE_CURVE('',#2811,#2811,#2497,.T.);
#3547=EDGE_CURVE('',#2812,#2812,#2498,.T.);
#3548=EDGE_CURVE('',#2813,#2813,#2499,.T.);
#3549=EDGE_CURVE('',#2814,#2815,#1772,.T.);
#3550=EDGE_CURVE('',#2814,#2816,#1773,.T.);
#3551=EDGE_CURVE('',#2816,#2817,#1774,.T.);
#3552=EDGE_CURVE('',#2815,#2817,#1775,.T.);
#3553=EDGE_CURVE('',#2818,#2814,#1776,.T.);
#3554=EDGE_CURVE('',#2818,#2819,#1777,.T.);
#3555=EDGE_CURVE('',#2819,#2816,#1778,.T.);
#3556=EDGE_CURVE('',#2820,#2818,#1779,.T.);
#3557=EDGE_CURVE('',#2820,#2821,#1780,.T.);
#3558=EDGE_CURVE('',#2821,#2819,#1781,.T.);
#3559=EDGE_CURVE('',#2822,#2820,#1782,.T.);
#3560=EDGE_CURVE('',#2822,#2823,#1783,.T.);
#3561=EDGE_CURVE('',#2823,#2821,#1784,.T.);
#3562=EDGE_CURVE('',#2824,#2822,#1785,.T.);
#3563=EDGE_CURVE('',#2824,#2825,#1786,.T.);
#3564=EDGE_CURVE('',#2825,#2823,#1787,.T.);
#3565=EDGE_CURVE('',#2815,#2824,#1788,.T.);
#3566=EDGE_CURVE('',#2817,#2825,#1789,.T.);
#3567=EDGE_CURVE('',#2826,#2826,#2500,.T.);
#3568=EDGE_CURVE('',#2827,#2828,#1790,.T.);
#3569=EDGE_CURVE('',#2827,#2829,#1791,.T.);
#3570=EDGE_CURVE('',#2829,#2830,#1792,.T.);
#3571=EDGE_CURVE('',#2828,#2830,#1793,.T.);
#3572=EDGE_CURVE('',#2831,#2827,#1794,.T.);
#3573=EDGE_CURVE('',#2831,#2832,#1795,.T.);
#3574=EDGE_CURVE('',#2832,#2829,#1796,.T.);
#3575=EDGE_CURVE('',#2833,#2831,#1797,.T.);
#3576=EDGE_CURVE('',#2833,#2834,#1798,.T.);
#3577=EDGE_CURVE('',#2834,#2832,#1799,.T.);
#3578=EDGE_CURVE('',#2835,#2833,#1800,.T.);
#3579=EDGE_CURVE('',#2835,#2836,#1801,.T.);
#3580=EDGE_CURVE('',#2836,#2834,#1802,.T.);
#3581=EDGE_CURVE('',#2837,#2835,#1803,.T.);
#3582=EDGE_CURVE('',#2837,#2838,#1804,.T.);
#3583=EDGE_CURVE('',#2838,#2836,#1805,.T.);
#3584=EDGE_CURVE('',#2828,#2837,#1806,.T.);
#3585=EDGE_CURVE('',#2830,#2838,#1807,.T.);
#3586=EDGE_CURVE('',#2839,#2839,#2501,.T.);
#3587=EDGE_CURVE('',#2840,#2840,#2502,.T.);
#3588=EDGE_CURVE('',#2840,#2811,#1808,.T.);
#3589=EDGE_CURVE('',#2841,#2841,#2503,.T.);
#3590=EDGE_CURVE('',#2841,#2842,#1809,.T.);
#3591=EDGE_CURVE('',#2842,#2842,#2504,.T.);
#3592=EDGE_CURVE('',#2843,#2843,#2505,.T.);
#3593=EDGE_CURVE('',#2843,#2844,#1810,.T.);
#3594=EDGE_CURVE('',#2844,#2844,#2506,.T.);
#3595=EDGE_CURVE('',#2845,#2845,#2507,.T.);
#3596=EDGE_CURVE('',#2845,#2812,#1811,.T.);
#3597=EDGE_CURVE('',#2839,#2846,#1812,.T.);
#3598=EDGE_CURVE('',#2846,#2846,#2508,.T.);
#3599=EDGE_CURVE('',#2826,#2847,#1813,.T.);
#3600=EDGE_CURVE('',#2847,#2847,#2509,.T.);
#3601=EDGE_CURVE('',#2848,#2849,#1814,.T.);
#3602=EDGE_CURVE('',#2850,#2848,#1815,.T.);
#3603=EDGE_CURVE('',#2851,#2850,#1816,.T.);
#3604=EDGE_CURVE('',#2851,#2849,#1817,.T.);
#3605=EDGE_CURVE('',#2852,#2853,#1818,.T.);
#3606=EDGE_CURVE('',#2852,#2854,#1819,.T.);
#3607=EDGE_CURVE('',#2855,#2854,#1820,.T.);
#3608=EDGE_CURVE('',#2853,#2855,#1821,.T.);
#3609=EDGE_CURVE('',#2856,#2857,#1822,.T.);
#3610=EDGE_CURVE('',#2856,#2858,#1823,.T.);
#3611=EDGE_CURVE('',#2859,#2858,#1824,.T.);
#3612=EDGE_CURVE('',#2857,#2859,#1825,.T.);
#3613=EDGE_CURVE('',#2860,#2861,#1826,.T.);
#3614=EDGE_CURVE('',#2860,#2862,#1827,.T.);
#3615=EDGE_CURVE('',#2863,#2862,#1828,.T.);
#3616=EDGE_CURVE('',#2861,#2863,#1829,.T.);
#3617=EDGE_CURVE('',#2864,#2865,#1830,.T.);
#3618=EDGE_CURVE('',#2864,#2866,#1831,.T.);
#3619=EDGE_CURVE('',#2867,#2866,#1832,.T.);
#3620=EDGE_CURVE('',#2865,#2867,#1833,.T.);
#3621=EDGE_CURVE('',#2868,#2869,#1834,.T.);
#3622=EDGE_CURVE('',#2870,#2868,#1835,.T.);
#3623=EDGE_CURVE('',#2871,#2870,#1836,.T.);
#3624=EDGE_CURVE('',#2871,#2869,#1837,.T.);
#3625=EDGE_CURVE('',#2872,#2873,#1838,.T.);
#3626=EDGE_CURVE('',#2874,#2872,#1839,.T.);
#3627=EDGE_CURVE('',#2875,#2874,#1840,.T.);
#3628=EDGE_CURVE('',#2875,#2873,#1841,.T.);
#3629=EDGE_CURVE('',#2876,#2876,#2510,.T.);
#3630=EDGE_CURVE('',#2877,#2877,#2511,.T.);
#3631=EDGE_CURVE('',#2849,#2864,#1842,.T.);
#3632=EDGE_CURVE('',#2866,#2851,#1843,.T.);
#3633=EDGE_CURVE('',#2869,#2852,#1844,.T.);
#3634=EDGE_CURVE('',#2854,#2871,#1845,.T.);
#3635=EDGE_CURVE('',#2873,#2856,#1846,.T.);
#3636=EDGE_CURVE('',#2858,#2875,#1847,.T.);
#3637=EDGE_CURVE('',#2878,#2860,#1848,.T.);
#3638=EDGE_CURVE('',#2879,#2878,#1849,.T.);
#3639=EDGE_CURVE('',#2862,#2879,#1850,.T.);
#3640=EDGE_CURVE('',#2880,#2878,#1851,.T.);
#3641=EDGE_CURVE('',#2881,#2880,#1852,.T.);
#3642=EDGE_CURVE('',#2879,#2881,#1853,.T.);
#3643=EDGE_CURVE('',#2882,#2883,#1854,.T.);
#3644=EDGE_CURVE('',#2884,#2883,#288,.T.);
#3645=EDGE_CURVE('',#2810,#2884,#289,.T.);
#3646=EDGE_CURVE('',#2882,#2807,#290,.T.);
#3647=EDGE_CURVE('',#2881,#2885,#1855,.T.);
#3648=EDGE_CURVE('',#2806,#2885,#291,.T.);
#3649=EDGE_CURVE('',#2886,#2809,#292,.T.);
#3650=EDGE_CURVE('',#2887,#2886,#293,.T.);
#3651=EDGE_CURVE('',#2887,#2863,#1856,.T.);
#3652=EDGE_CURVE('',#2874,#2888,#1857,.T.);
#3653=EDGE_CURVE('',#2889,#2888,#294,.T.);
#3654=EDGE_CURVE('',#2890,#2889,#295,.T.);
#3655=EDGE_CURVE('',#2891,#2890,#1858,.T.);
#3656=EDGE_CURVE('',#2892,#2891,#296,.T.);
#3657=EDGE_CURVE('',#2893,#2892,#297,.T.);
#3658=EDGE_CURVE('',#2893,#2859,#1859,.T.);
#3659=EDGE_CURVE('',#2870,#2894,#1860,.T.);
#3660=EDGE_CURVE('',#2802,#2894,#298,.T.);
#3661=EDGE_CURVE('',#2895,#2801,#1861,.T.);
#3662=EDGE_CURVE('',#2896,#2895,#299,.T.);
#3663=EDGE_CURVE('',#2897,#2896,#300,.T.);
#3664=EDGE_CURVE('',#2897,#2855,#1862,.T.);
#3665=EDGE_CURVE('',#2898,#2865,#1863,.T.);
#3666=EDGE_CURVE('',#2898,#2899,#301,.T.);
#3667=EDGE_CURVE('',#2899,#2900,#1864,.T.);
#3668=EDGE_CURVE('',#2900,#2901,#302,.T.);
#3669=EDGE_CURVE('',#2848,#2901,#1865,.T.);
#3670=EDGE_CURVE('',#2887,#2883,#303,.T.);
#3671=EDGE_CURVE('',#2882,#2885,#304,.T.);
#3672=EDGE_CURVE('',#2902,#2880,#1866,.T.);
#3673=EDGE_CURVE('',#2902,#2888,#305,.T.);
#3674=EDGE_CURVE('',#2903,#2872,#1867,.T.);
#3675=EDGE_CURVE('',#2903,#2894,#306,.T.);
#3676=EDGE_CURVE('',#2904,#2868,#1868,.T.);
#3677=EDGE_CURVE('',#2904,#2905,#307,.T.);
#3678=EDGE_CURVE('',#2905,#2898,#308,.T.);
#3679=EDGE_CURVE('',#2867,#2906,#1869,.T.);
#3680=EDGE_CURVE('',#2907,#2906,#309,.T.);
#3681=EDGE_CURVE('',#2907,#2908,#310,.T.);
#3682=EDGE_CURVE('',#2909,#2908,#311,.T.);
#3683=EDGE_CURVE('',#2909,#2910,#1870,.T.);
#3684=EDGE_CURVE('',#2911,#2910,#312,.T.);
#3685=EDGE_CURVE('',#2911,#2912,#313,.T.);
#3686=EDGE_CURVE('',#2913,#2912,#314,.T.);
#3687=EDGE_CURVE('',#2913,#2850,#1871,.T.);
#3688=EDGE_CURVE('',#2901,#2914,#315,.T.);
#3689=EDGE_CURVE('',#2914,#2915,#316,.T.);
#3690=EDGE_CURVE('',#2853,#2915,#1872,.T.);
#3691=EDGE_CURVE('',#2897,#2916,#317,.T.);
#3692=EDGE_CURVE('',#2857,#2916,#1873,.T.);
#3693=EDGE_CURVE('',#2893,#2917,#318,.T.);
#3694=EDGE_CURVE('',#2861,#2917,#1874,.T.);
#3695=EDGE_CURVE('',#2918,#2919,#319,.T.);
#3696=EDGE_CURVE('',#2919,#2920,#320,.T.);
#3697=EDGE_CURVE('',#2920,#2921,#1875,.T.);
#3698=EDGE_CURVE('',#2921,#2922,#321,.T.);
#3699=EDGE_CURVE('',#2922,#2923,#322,.T.);
#3700=EDGE_CURVE('',#2918,#2923,#1876,.T.);
#3701=EDGE_CURVE('',#2813,#2877,#1877,.T.);
#3702=EDGE_CURVE('',#2924,#2924,#2512,.T.);
#3703=EDGE_CURVE('',#2924,#2876,#1878,.T.);
#3704=EDGE_CURVE('',#2918,#2925,#323,.T.);
#3705=EDGE_CURVE('',#2926,#2923,#324,.T.);
#3706=EDGE_CURVE('',#2927,#2926,#325,.T.);
#3707=EDGE_CURVE('',#2928,#2927,#1879,.T.);
#3708=EDGE_CURVE('',#2925,#2928,#326,.T.);
#3709=EDGE_CURVE('',#2886,#2884,#327,.T.);
#3710=EDGE_CURVE('',#2925,#2929,#328,.T.);
#3711=EDGE_CURVE('',#2929,#2919,#329,.T.);
#3712=EDGE_CURVE('',#2930,#2928,#330,.T.);
#3713=EDGE_CURVE('',#2929,#2930,#2513,.F.);
#3714=EDGE_CURVE('',#2927,#2931,#331,.T.);
#3715=EDGE_CURVE('',#2931,#2930,#1880,.T.);
#3716=EDGE_CURVE('',#2922,#2932,#332,.T.);
#3717=EDGE_CURVE('',#2932,#2926,#333,.T.);
#3718=EDGE_CURVE('',#2933,#2917,#334,.T.);
#3719=EDGE_CURVE('',#2934,#2933,#335,.T.);
#3720=EDGE_CURVE('',#2935,#2934,#1881,.T.);
#3721=EDGE_CURVE('',#2936,#2935,#336,.T.);
#3722=EDGE_CURVE('',#2902,#2936,#337,.T.);
#3723=EDGE_CURVE('',#2892,#2933,#338,.T.);
#3724=EDGE_CURVE('',#2934,#2891,#339,.T.);
#3725=EDGE_CURVE('',#2890,#2935,#340,.T.);
#3726=EDGE_CURVE('',#2936,#2889,#341,.T.);
#3727=EDGE_CURVE('',#2937,#2916,#342,.T.);
#3728=EDGE_CURVE('',#2938,#2937,#343,.T.);
#3729=EDGE_CURVE('',#2804,#2938,#1882,.T.);
#3730=EDGE_CURVE('',#2903,#2803,#344,.T.);
#3731=EDGE_CURVE('',#2896,#2937,#345,.T.);
#3732=EDGE_CURVE('',#2938,#2798,#346,.T.);
#3733=EDGE_CURVE('',#2797,#2895,#347,.T.);
#3734=EDGE_CURVE('',#2939,#2915,#348,.T.);
#3735=EDGE_CURVE('',#2940,#2939,#349,.T.);
#3736=EDGE_CURVE('',#2941,#2940,#1883,.T.);
#3737=EDGE_CURVE('',#2942,#2941,#350,.T.);
#3738=EDGE_CURVE('',#2904,#2942,#351,.T.);
#3739=EDGE_CURVE('',#2914,#2943,#352,.T.);
#3740=EDGE_CURVE('',#2943,#2939,#353,.T.);
#3741=EDGE_CURVE('',#2944,#2943,#2514,.F.);
#3742=EDGE_CURVE('',#2940,#2944,#354,.T.);
#3743=EDGE_CURVE('',#2944,#2945,#1884,.T.);
#3744=EDGE_CURVE('',#2945,#2941,#355,.T.);
#3745=EDGE_CURVE('',#2942,#2946,#356,.T.);
#3746=EDGE_CURVE('',#2946,#2905,#357,.T.);
#3747=EDGE_CURVE('',#2946,#2945,#2515,.F.);
#3748=EDGE_CURVE('',#2945,#2899,#2516,.F.);
#3749=EDGE_CURVE('',#2899,#2946,#2517,.F.);
#3750=EDGE_CURVE('',#2931,#2932,#2518,.F.);
#3751=EDGE_CURVE('',#2932,#2947,#2519,.F.);
#3752=EDGE_CURVE('',#2947,#2931,#2520,.F.);
#3753=EDGE_CURVE('',#2943,#2900,#2521,.F.);
#3754=EDGE_CURVE('',#2900,#2944,#2522,.F.);
#3755=EDGE_CURVE('',#2948,#2929,#2523,.F.);
#3756=EDGE_CURVE('',#2930,#2948,#2524,.F.);
#3757=EDGE_CURVE('',#2948,#2947,#1885,.T.);
#3758=EDGE_CURVE('',#2920,#2948,#358,.T.);
#3759=EDGE_CURVE('',#2947,#2921,#359,.T.);
#3760=EDGE_CURVE('',#2949,#2950,#2525,.F.);
#3761=EDGE_CURVE('',#2951,#2949,#2526,.F.);
#3762=EDGE_CURVE('',#2950,#2951,#2527,.F.);
#3763=EDGE_CURVE('',#2952,#2953,#2528,.F.);
#3764=EDGE_CURVE('',#2954,#2952,#2529,.F.);
#3765=EDGE_CURVE('',#2953,#2954,#2530,.F.);
#3766=EDGE_CURVE('',#2955,#2956,#2531,.F.);
#3767=EDGE_CURVE('',#2957,#2955,#2532,.F.);
#3768=EDGE_CURVE('',#2956,#2957,#2533,.F.);
#3769=EDGE_CURVE('',#2950,#2957,#1886,.T.);
#3770=EDGE_CURVE('',#2955,#2949,#1887,.T.);
#3771=EDGE_CURVE('',#2912,#2956,#360,.T.);
#3772=EDGE_CURVE('',#2957,#2913,#361,.T.);
#3773=EDGE_CURVE('',#2958,#2959,#2534,.F.);
#3774=EDGE_CURVE('',#2960,#2958,#2535,.F.);
#3775=EDGE_CURVE('',#2959,#2960,#2536,.F.);
#3776=EDGE_CURVE('',#2958,#2954,#1888,.T.);
#3777=EDGE_CURVE('',#2952,#2960,#1889,.T.);
#3778=EDGE_CURVE('',#2956,#2959,#362,.T.);
#3779=EDGE_CURVE('',#2960,#2955,#363,.T.);
#3780=EDGE_CURVE('',#2910,#2958,#364,.T.);
#3781=EDGE_CURVE('',#2959,#2911,#365,.T.);
#3782=EDGE_CURVE('',#2908,#2953,#366,.T.);
#3783=EDGE_CURVE('',#2954,#2909,#367,.T.);
#3784=EDGE_CURVE('',#2953,#2951,#368,.T.);
#3785=EDGE_CURVE('',#2949,#2952,#369,.T.);
#3786=EDGE_CURVE('',#2906,#2950,#370,.T.);
#3787=EDGE_CURVE('',#2951,#2907,#371,.T.);
#4802=ORIENTED_EDGE('',*,*,#3524,.F.);
#4803=ORIENTED_EDGE('',*,*,#3525,.T.);
#4804=ORIENTED_EDGE('',*,*,#3526,.F.);
#4805=ORIENTED_EDGE('',*,*,#3527,.T.);
#4806=ORIENTED_EDGE('',*,*,#3528,.F.);
#4807=ORIENTED_EDGE('',*,*,#3529,.T.);
#4808=ORIENTED_EDGE('',*,*,#3530,.F.);
#4809=ORIENTED_EDGE('',*,*,#3531,.T.);
#4810=ORIENTED_EDGE('',*,*,#3526,.T.);
#4811=ORIENTED_EDGE('',*,*,#3532,.F.);
#4812=ORIENTED_EDGE('',*,*,#3533,.T.);
#4813=ORIENTED_EDGE('',*,*,#3534,.F.);
#4814=ORIENTED_EDGE('',*,*,#3535,.T.);
#4815=ORIENTED_EDGE('',*,*,#3536,.F.);
#4816=ORIENTED_EDGE('',*,*,#3530,.T.);
#4817=ORIENTED_EDGE('',*,*,#3537,.F.);
#4818=ORIENTED_EDGE('',*,*,#3538,.T.);
#4819=ORIENTED_EDGE('',*,*,#3539,.F.);
#4820=ORIENTED_EDGE('',*,*,#3540,.T.);
#4821=ORIENTED_EDGE('',*,*,#3541,.F.);
#4822=ORIENTED_EDGE('',*,*,#3542,.T.);
#4823=ORIENTED_EDGE('',*,*,#3543,.T.);
#4824=ORIENTED_EDGE('',*,*,#3537,.T.);
#4825=ORIENTED_EDGE('',*,*,#3531,.F.);
#4826=ORIENTED_EDGE('',*,*,#3541,.T.);
#4827=ORIENTED_EDGE('',*,*,#3544,.T.);
#4828=ORIENTED_EDGE('',*,*,#3545,.T.);
#4829=ORIENTED_EDGE('',*,*,#3525,.F.);
#4830=ORIENTED_EDGE('',*,*,#3546,.T.);
#4831=ORIENTED_EDGE('',*,*,#3547,.T.);
#4832=ORIENTED_EDGE('',*,*,#3548,.T.);
#4833=ORIENTED_EDGE('',*,*,#3549,.F.);
#4834=ORIENTED_EDGE('',*,*,#3550,.T.);
#4835=ORIENTED_EDGE('',*,*,#3551,.T.);
#4836=ORIENTED_EDGE('',*,*,#3552,.F.);
#4837=ORIENTED_EDGE('',*,*,#3553,.F.);
#4838=ORIENTED_EDGE('',*,*,#3554,.T.);
#4839=ORIENTED_EDGE('',*,*,#3555,.T.);
#4840=ORIENTED_EDGE('',*,*,#3550,.F.);
#4841=ORIENTED_EDGE('',*,*,#3556,.F.);
#4842=ORIENTED_EDGE('',*,*,#3557,.T.);
#4843=ORIENTED_EDGE('',*,*,#3558,.T.);
#4844=ORIENTED_EDGE('',*,*,#3554,.F.);
#4845=ORIENTED_EDGE('',*,*,#3559,.F.);
#4846=ORIENTED_EDGE('',*,*,#3560,.T.);
#4847=ORIENTED_EDGE('',*,*,#3561,.T.);
#4848=ORIENTED_EDGE('',*,*,#3557,.F.);
#4849=ORIENTED_EDGE('',*,*,#3562,.F.);
#4850=ORIENTED_EDGE('',*,*,#3563,.T.);
#4851=ORIENTED_EDGE('',*,*,#3564,.T.);
#4852=ORIENTED_EDGE('',*,*,#3560,.F.);
#4853=ORIENTED_EDGE('',*,*,#3565,.F.);
#4854=ORIENTED_EDGE('',*,*,#3552,.T.);
#4855=ORIENTED_EDGE('',*,*,#3566,.T.);
#4856=ORIENTED_EDGE('',*,*,#3563,.F.);
#4857=ORIENTED_EDGE('',*,*,#3566,.F.);
#4858=ORIENTED_EDGE('',*,*,#3551,.F.);
#4859=ORIENTED_EDGE('',*,*,#3555,.F.);
#4860=ORIENTED_EDGE('',*,*,#3558,.F.);
#4861=ORIENTED_EDGE('',*,*,#3561,.F.);
#4862=ORIENTED_EDGE('',*,*,#3564,.F.);
#4863=ORIENTED_EDGE('',*,*,#3567,.F.);
#4864=ORIENTED_EDGE('',*,*,#3568,.F.);
#4865=ORIENTED_EDGE('',*,*,#3569,.T.);
#4866=ORIENTED_EDGE('',*,*,#3570,.T.);
#4867=ORIENTED_EDGE('',*,*,#3571,.F.);
#4868=ORIENTED_EDGE('',*,*,#3572,.F.);
#4869=ORIENTED_EDGE('',*,*,#3573,.T.);
#4870=ORIENTED_EDGE('',*,*,#3574,.T.);
#4871=ORIENTED_EDGE('',*,*,#3569,.F.);
#4872=ORIENTED_EDGE('',*,*,#3575,.F.);
#4873=ORIENTED_EDGE('',*,*,#3576,.T.);
#4874=ORIENTED_EDGE('',*,*,#3577,.T.);
#4875=ORIENTED_EDGE('',*,*,#3573,.F.);
#4876=ORIENTED_EDGE('',*,*,#3578,.F.);
#4877=ORIENTED_EDGE('',*,*,#3579,.T.);
#4878=ORIENTED_EDGE('',*,*,#3580,.T.);
#4879=ORIENTED_EDGE('',*,*,#3576,.F.);
#4880=ORIENTED_EDGE('',*,*,#3581,.F.);
#4881=ORIENTED_EDGE('',*,*,#3582,.T.);
#4882=ORIENTED_EDGE('',*,*,#3583,.T.);
#4883=ORIENTED_EDGE('',*,*,#3579,.F.);
#4884=ORIENTED_EDGE('',*,*,#3584,.F.);
#4885=ORIENTED_EDGE('',*,*,#3571,.T.);
#4886=ORIENTED_EDGE('',*,*,#3585,.T.);
#4887=ORIENTED_EDGE('',*,*,#3582,.F.);
#4888=ORIENTED_EDGE('',*,*,#3585,.F.);
#4889=ORIENTED_EDGE('',*,*,#3570,.F.);
#4890=ORIENTED_EDGE('',*,*,#3574,.F.);
#4891=ORIENTED_EDGE('',*,*,#3577,.F.);
#4892=ORIENTED_EDGE('',*,*,#3580,.F.);
#4893=ORIENTED_EDGE('',*,*,#3583,.F.);
#4894=ORIENTED_EDGE('',*,*,#3586,.F.);
#4895=ORIENTED_EDGE('',*,*,#3587,.F.);
#4896=ORIENTED_EDGE('',*,*,#3588,.T.);
#4897=ORIENTED_EDGE('',*,*,#3546,.F.);
#4898=ORIENTED_EDGE('',*,*,#3588,.F.);
#4899=ORIENTED_EDGE('',*,*,#3589,.F.);
#4900=ORIENTED_EDGE('',*,*,#3590,.T.);
#4901=ORIENTED_EDGE('',*,*,#3591,.F.);
#4902=ORIENTED_EDGE('',*,*,#3590,.F.);
#4903=ORIENTED_EDGE('',*,*,#3592,.F.);
#4904=ORIENTED_EDGE('',*,*,#3593,.T.);
#4905=ORIENTED_EDGE('',*,*,#3594,.F.);
#4906=ORIENTED_EDGE('',*,*,#3593,.F.);
#4907=ORIENTED_EDGE('',*,*,#3595,.F.);
#4908=ORIENTED_EDGE('',*,*,#3596,.T.);
#4909=ORIENTED_EDGE('',*,*,#3547,.F.);
#4910=ORIENTED_EDGE('',*,*,#3596,.F.);
#4911=ORIENTED_EDGE('',*,*,#3586,.T.);
#4912=ORIENTED_EDGE('',*,*,#3597,.T.);
#4913=ORIENTED_EDGE('',*,*,#3598,.F.);
#4914=ORIENTED_EDGE('',*,*,#3597,.F.);
#4915=ORIENTED_EDGE('',*,*,#3567,.T.);
#4916=ORIENTED_EDGE('',*,*,#3599,.T.);
#4917=ORIENTED_EDGE('',*,*,#3600,.F.);
#4918=ORIENTED_EDGE('',*,*,#3599,.F.);
#4919=ORIENTED_EDGE('',*,*,#3601,.F.);
#4920=ORIENTED_EDGE('',*,*,#3602,.F.);
#4921=ORIENTED_EDGE('',*,*,#3603,.F.);
#4922=ORIENTED_EDGE('',*,*,#3604,.T.);
#4923=ORIENTED_EDGE('',*,*,#3605,.F.);
#4924=ORIENTED_EDGE('',*,*,#3606,.T.);
#4925=ORIENTED_EDGE('',*,*,#3607,.F.);
#4926=ORIENTED_EDGE('',*,*,#3608,.F.);
#4927=ORIENTED_EDGE('',*,*,#3609,.F.);
#4928=ORIENTED_EDGE('',*,*,#3610,.T.);
#4929=ORIENTED_EDGE('',*,*,#3611,.F.);
#4930=ORIENTED_EDGE('',*,*,#3612,.F.);
#4931=ORIENTED_EDGE('',*,*,#3613,.F.);
#4932=ORIENTED_EDGE('',*,*,#3614,.T.);
#4933=ORIENTED_EDGE('',*,*,#3615,.F.);
#4934=ORIENTED_EDGE('',*,*,#3616,.F.);
#4935=ORIENTED_EDGE('',*,*,#3617,.F.);
#4936=ORIENTED_EDGE('',*,*,#3618,.T.);
#4937=ORIENTED_EDGE('',*,*,#3619,.F.);
#4938=ORIENTED_EDGE('',*,*,#3620,.F.);
#4939=ORIENTED_EDGE('',*,*,#3621,.F.);
#4940=ORIENTED_EDGE('',*,*,#3622,.F.);
#4941=ORIENTED_EDGE('',*,*,#3623,.F.);
#4942=ORIENTED_EDGE('',*,*,#3624,.T.);
#4943=ORIENTED_EDGE('',*,*,#3625,.F.);
#4944=ORIENTED_EDGE('',*,*,#3626,.F.);
#4945=ORIENTED_EDGE('',*,*,#3627,.F.);
#4946=ORIENTED_EDGE('',*,*,#3628,.T.);
#4947=ORIENTED_EDGE('',*,*,#3629,.F.);
#4948=ORIENTED_EDGE('',*,*,#3598,.T.);
#4949=ORIENTED_EDGE('',*,*,#3630,.F.);
#4950=ORIENTED_EDGE('',*,*,#3600,.T.);
#4951=ORIENTED_EDGE('',*,*,#3631,.F.);
#4952=ORIENTED_EDGE('',*,*,#3604,.F.);
#4953=ORIENTED_EDGE('',*,*,#3632,.F.);
#4954=ORIENTED_EDGE('',*,*,#3618,.F.);
#4955=ORIENTED_EDGE('',*,*,#3633,.F.);
#4956=ORIENTED_EDGE('',*,*,#3624,.F.);
#4957=ORIENTED_EDGE('',*,*,#3634,.F.);
#4958=ORIENTED_EDGE('',*,*,#3606,.F.);
#4959=ORIENTED_EDGE('',*,*,#3635,.F.);
#4960=ORIENTED_EDGE('',*,*,#3628,.F.);
#4961=ORIENTED_EDGE('',*,*,#3636,.F.);
#4962=ORIENTED_EDGE('',*,*,#3610,.F.);
#4963=ORIENTED_EDGE('',*,*,#3637,.F.);
#4964=ORIENTED_EDGE('',*,*,#3638,.F.);
#4965=ORIENTED_EDGE('',*,*,#3639,.F.);
#4966=ORIENTED_EDGE('',*,*,#3614,.F.);
#4967=ORIENTED_EDGE('',*,*,#3640,.F.);
#4968=ORIENTED_EDGE('',*,*,#3641,.F.);
#4969=ORIENTED_EDGE('',*,*,#3642,.F.);
#4970=ORIENTED_EDGE('',*,*,#3638,.T.);
#4971=ORIENTED_EDGE('',*,*,#3643,.T.);
#4972=ORIENTED_EDGE('',*,*,#3644,.F.);
#4973=ORIENTED_EDGE('',*,*,#3645,.F.);
#4974=ORIENTED_EDGE('',*,*,#3544,.F.);
#4975=ORIENTED_EDGE('',*,*,#3540,.F.);
#4976=ORIENTED_EDGE('',*,*,#3646,.F.);
#4977=ORIENTED_EDGE('',*,*,#3615,.T.);
#4978=ORIENTED_EDGE('',*,*,#3639,.T.);
#4979=ORIENTED_EDGE('',*,*,#3642,.T.);
#4980=ORIENTED_EDGE('',*,*,#3647,.T.);
#4981=ORIENTED_EDGE('',*,*,#3648,.F.);
#4982=ORIENTED_EDGE('',*,*,#3538,.F.);
#4983=ORIENTED_EDGE('',*,*,#3543,.F.);
#4984=ORIENTED_EDGE('',*,*,#3649,.F.);
#4985=ORIENTED_EDGE('',*,*,#3650,.F.);
#4986=ORIENTED_EDGE('',*,*,#3651,.T.);
#4987=ORIENTED_EDGE('',*,*,#3611,.T.);
#4988=ORIENTED_EDGE('',*,*,#3636,.T.);
#4989=ORIENTED_EDGE('',*,*,#3627,.T.);
#4990=ORIENTED_EDGE('',*,*,#3652,.T.);
#4991=ORIENTED_EDGE('',*,*,#3653,.F.);
#4992=ORIENTED_EDGE('',*,*,#3654,.F.);
#4993=ORIENTED_EDGE('',*,*,#3655,.F.);
#4994=ORIENTED_EDGE('',*,*,#3656,.F.);
#4995=ORIENTED_EDGE('',*,*,#3657,.F.);
#4996=ORIENTED_EDGE('',*,*,#3658,.T.);
#4997=ORIENTED_EDGE('',*,*,#3607,.T.);
#4998=ORIENTED_EDGE('',*,*,#3634,.T.);
#4999=ORIENTED_EDGE('',*,*,#3623,.T.);
#5000=ORIENTED_EDGE('',*,*,#3659,.T.);
#5001=ORIENTED_EDGE('',*,*,#3660,.F.);
#5002=ORIENTED_EDGE('',*,*,#3533,.F.);
#5003=ORIENTED_EDGE('',*,*,#3661,.F.);
#5004=ORIENTED_EDGE('',*,*,#3662,.F.);
#5005=ORIENTED_EDGE('',*,*,#3663,.F.);
#5006=ORIENTED_EDGE('',*,*,#3664,.T.);
#5007=ORIENTED_EDGE('',*,*,#3601,.T.);
#5008=ORIENTED_EDGE('',*,*,#3631,.T.);
#5009=ORIENTED_EDGE('',*,*,#3617,.T.);
#5010=ORIENTED_EDGE('',*,*,#3665,.F.);
#5011=ORIENTED_EDGE('',*,*,#3666,.T.);
#5012=ORIENTED_EDGE('',*,*,#3667,.T.);
#5013=ORIENTED_EDGE('',*,*,#3668,.T.);
#5014=ORIENTED_EDGE('',*,*,#3669,.F.);
#5015=ORIENTED_EDGE('',*,*,#3616,.T.);
#5016=ORIENTED_EDGE('',*,*,#3651,.F.);
#5017=ORIENTED_EDGE('',*,*,#3670,.T.);
#5018=ORIENTED_EDGE('',*,*,#3643,.F.);
#5019=ORIENTED_EDGE('',*,*,#3671,.T.);
#5020=ORIENTED_EDGE('',*,*,#3647,.F.);
#5021=ORIENTED_EDGE('',*,*,#3641,.T.);
#5022=ORIENTED_EDGE('',*,*,#3672,.F.);
#5023=ORIENTED_EDGE('',*,*,#3673,.T.);
#5024=ORIENTED_EDGE('',*,*,#3652,.F.);
#5025=ORIENTED_EDGE('',*,*,#3626,.T.);
#5026=ORIENTED_EDGE('',*,*,#3674,.F.);
#5027=ORIENTED_EDGE('',*,*,#3675,.T.);
#5028=ORIENTED_EDGE('',*,*,#3659,.F.);
#5029=ORIENTED_EDGE('',*,*,#3622,.T.);
#5030=ORIENTED_EDGE('',*,*,#3676,.F.);
#5031=ORIENTED_EDGE('',*,*,#3677,.T.);
#5032=ORIENTED_EDGE('',*,*,#3678,.T.);
#5033=ORIENTED_EDGE('',*,*,#3665,.T.);
#5034=ORIENTED_EDGE('',*,*,#3620,.T.);
#5035=ORIENTED_EDGE('',*,*,#3679,.T.);
#5036=ORIENTED_EDGE('',*,*,#3680,.F.);
#5037=ORIENTED_EDGE('',*,*,#3681,.T.);
#5038=ORIENTED_EDGE('',*,*,#3682,.F.);
#5039=ORIENTED_EDGE('',*,*,#3683,.T.);
#5040=ORIENTED_EDGE('',*,*,#3684,.F.);
#5041=ORIENTED_EDGE('',*,*,#3685,.T.);
#5042=ORIENTED_EDGE('',*,*,#3686,.F.);
#5043=ORIENTED_EDGE('',*,*,#3687,.T.);
#5044=ORIENTED_EDGE('',*,*,#3602,.T.);
#5045=ORIENTED_EDGE('',*,*,#3669,.T.);
#5046=ORIENTED_EDGE('',*,*,#3688,.T.);
#5047=ORIENTED_EDGE('',*,*,#3689,.T.);
#5048=ORIENTED_EDGE('',*,*,#3690,.F.);
#5049=ORIENTED_EDGE('',*,*,#3608,.T.);
#5050=ORIENTED_EDGE('',*,*,#3664,.F.);
#5051=ORIENTED_EDGE('',*,*,#3691,.T.);
#5052=ORIENTED_EDGE('',*,*,#3692,.F.);
#5053=ORIENTED_EDGE('',*,*,#3612,.T.);
#5054=ORIENTED_EDGE('',*,*,#3658,.F.);
#5055=ORIENTED_EDGE('',*,*,#3693,.T.);
#5056=ORIENTED_EDGE('',*,*,#3694,.F.);
#5057=ORIENTED_EDGE('',*,*,#3695,.T.);
#5058=ORIENTED_EDGE('',*,*,#3696,.T.);
#5059=ORIENTED_EDGE('',*,*,#3697,.T.);
#5060=ORIENTED_EDGE('',*,*,#3698,.T.);
#5061=ORIENTED_EDGE('',*,*,#3699,.T.);
#5062=ORIENTED_EDGE('',*,*,#3700,.F.);
#5063=ORIENTED_EDGE('',*,*,#3548,.F.);
#5064=ORIENTED_EDGE('',*,*,#3701,.T.);
#5065=ORIENTED_EDGE('',*,*,#3630,.T.);
#5066=ORIENTED_EDGE('',*,*,#3701,.F.);
#5067=ORIENTED_EDGE('',*,*,#3702,.F.);
#5068=ORIENTED_EDGE('',*,*,#3703,.T.);
#5069=ORIENTED_EDGE('',*,*,#3629,.T.);
#5070=ORIENTED_EDGE('',*,*,#3703,.F.);
#5071=ORIENTED_EDGE('',*,*,#3704,.F.);
#5072=ORIENTED_EDGE('',*,*,#3700,.T.);
#5073=ORIENTED_EDGE('',*,*,#3705,.F.);
#5074=ORIENTED_EDGE('',*,*,#3706,.F.);
#5075=ORIENTED_EDGE('',*,*,#3707,.F.);
#5076=ORIENTED_EDGE('',*,*,#3708,.F.);
#5077=ORIENTED_EDGE('',*,*,#3644,.T.);
#5078=ORIENTED_EDGE('',*,*,#3670,.F.);
#5079=ORIENTED_EDGE('',*,*,#3650,.T.);
#5080=ORIENTED_EDGE('',*,*,#3709,.T.);
#5081=ORIENTED_EDGE('',*,*,#3704,.T.);
#5082=ORIENTED_EDGE('',*,*,#3710,.T.);
#5083=ORIENTED_EDGE('',*,*,#3711,.T.);
#5084=ORIENTED_EDGE('',*,*,#3695,.F.);
#5085=ORIENTED_EDGE('',*,*,#3524,.T.);
#5086=ORIENTED_EDGE('',*,*,#3545,.F.);
#5087=ORIENTED_EDGE('',*,*,#3645,.T.);
#5088=ORIENTED_EDGE('',*,*,#3709,.F.);
#5089=ORIENTED_EDGE('',*,*,#3649,.T.);
#5090=ORIENTED_EDGE('',*,*,#3542,.F.);
#5091=ORIENTED_EDGE('',*,*,#3708,.T.);
#5092=ORIENTED_EDGE('',*,*,#3712,.F.);
#5093=ORIENTED_EDGE('',*,*,#3713,.F.);
#5094=ORIENTED_EDGE('',*,*,#3710,.F.);
#5095=ORIENTED_EDGE('',*,*,#3707,.T.);
#5096=ORIENTED_EDGE('',*,*,#3714,.T.);
#5097=ORIENTED_EDGE('',*,*,#3715,.T.);
#5098=ORIENTED_EDGE('',*,*,#3712,.T.);
#5099=ORIENTED_EDGE('',*,*,#3646,.T.);
#5100=ORIENTED_EDGE('',*,*,#3539,.T.);
#5101=ORIENTED_EDGE('',*,*,#3648,.T.);
#5102=ORIENTED_EDGE('',*,*,#3671,.F.);
#5103=ORIENTED_EDGE('',*,*,#3705,.T.);
#5104=ORIENTED_EDGE('',*,*,#3699,.F.);
#5105=ORIENTED_EDGE('',*,*,#3716,.T.);
#5106=ORIENTED_EDGE('',*,*,#3717,.T.);
#5107=ORIENTED_EDGE('',*,*,#3613,.T.);
#5108=ORIENTED_EDGE('',*,*,#3694,.T.);
#5109=ORIENTED_EDGE('',*,*,#3718,.F.);
#5110=ORIENTED_EDGE('',*,*,#3719,.F.);
#5111=ORIENTED_EDGE('',*,*,#3720,.F.);
#5112=ORIENTED_EDGE('',*,*,#3721,.F.);
#5113=ORIENTED_EDGE('',*,*,#3722,.F.);
#5114=ORIENTED_EDGE('',*,*,#3672,.T.);
#5115=ORIENTED_EDGE('',*,*,#3640,.T.);
#5116=ORIENTED_EDGE('',*,*,#3637,.T.);
#5117=ORIENTED_EDGE('',*,*,#3718,.T.);
#5118=ORIENTED_EDGE('',*,*,#3693,.F.);
#5119=ORIENTED_EDGE('',*,*,#3657,.T.);
#5120=ORIENTED_EDGE('',*,*,#3723,.T.);
#5121=ORIENTED_EDGE('',*,*,#3719,.T.);
#5122=ORIENTED_EDGE('',*,*,#3723,.F.);
#5123=ORIENTED_EDGE('',*,*,#3656,.T.);
#5124=ORIENTED_EDGE('',*,*,#3724,.F.);
#5125=ORIENTED_EDGE('',*,*,#3720,.T.);
#5126=ORIENTED_EDGE('',*,*,#3724,.T.);
#5127=ORIENTED_EDGE('',*,*,#3655,.T.);
#5128=ORIENTED_EDGE('',*,*,#3725,.T.);
#5129=ORIENTED_EDGE('',*,*,#3721,.T.);
#5130=ORIENTED_EDGE('',*,*,#3725,.F.);
#5131=ORIENTED_EDGE('',*,*,#3654,.T.);
#5132=ORIENTED_EDGE('',*,*,#3726,.F.);
#5133=ORIENTED_EDGE('',*,*,#3722,.T.);
#5134=ORIENTED_EDGE('',*,*,#3726,.T.);
#5135=ORIENTED_EDGE('',*,*,#3653,.T.);
#5136=ORIENTED_EDGE('',*,*,#3673,.F.);
#5137=ORIENTED_EDGE('',*,*,#3609,.T.);
#5138=ORIENTED_EDGE('',*,*,#3692,.T.);
#5139=ORIENTED_EDGE('',*,*,#3727,.F.);
#5140=ORIENTED_EDGE('',*,*,#3728,.F.);
#5141=ORIENTED_EDGE('',*,*,#3729,.F.);
#5142=ORIENTED_EDGE('',*,*,#3535,.F.);
#5143=ORIENTED_EDGE('',*,*,#3730,.F.);
#5144=ORIENTED_EDGE('',*,*,#3674,.T.);
#5145=ORIENTED_EDGE('',*,*,#3625,.T.);
#5146=ORIENTED_EDGE('',*,*,#3635,.T.);
#5147=ORIENTED_EDGE('',*,*,#3727,.T.);
#5148=ORIENTED_EDGE('',*,*,#3691,.F.);
#5149=ORIENTED_EDGE('',*,*,#3663,.T.);
#5150=ORIENTED_EDGE('',*,*,#3731,.T.);
#5151=ORIENTED_EDGE('',*,*,#3528,.T.);
#5152=ORIENTED_EDGE('',*,*,#3732,.F.);
#5153=ORIENTED_EDGE('',*,*,#3728,.T.);
#5154=ORIENTED_EDGE('',*,*,#3731,.F.);
#5155=ORIENTED_EDGE('',*,*,#3662,.T.);
#5156=ORIENTED_EDGE('',*,*,#3733,.F.);
#5157=ORIENTED_EDGE('',*,*,#3536,.T.);
#5158=ORIENTED_EDGE('',*,*,#3729,.T.);
#5159=ORIENTED_EDGE('',*,*,#3732,.T.);
#5160=ORIENTED_EDGE('',*,*,#3529,.F.);
#5161=ORIENTED_EDGE('',*,*,#3733,.T.);
#5162=ORIENTED_EDGE('',*,*,#3661,.T.);
#5163=ORIENTED_EDGE('',*,*,#3532,.T.);
#5164=ORIENTED_EDGE('',*,*,#3527,.F.);
#5165=ORIENTED_EDGE('',*,*,#3594,.T.);
#5166=ORIENTED_EDGE('',*,*,#3591,.T.);
#5167=ORIENTED_EDGE('',*,*,#3702,.T.);
#5168=ORIENTED_EDGE('',*,*,#3730,.T.);
#5169=ORIENTED_EDGE('',*,*,#3534,.T.);
#5170=ORIENTED_EDGE('',*,*,#3660,.T.);
#5171=ORIENTED_EDGE('',*,*,#3675,.F.);
#5172=ORIENTED_EDGE('',*,*,#3605,.T.);
#5173=ORIENTED_EDGE('',*,*,#3690,.T.);
#5174=ORIENTED_EDGE('',*,*,#3734,.F.);
#5175=ORIENTED_EDGE('',*,*,#3735,.F.);
#5176=ORIENTED_EDGE('',*,*,#3736,.F.);
#5177=ORIENTED_EDGE('',*,*,#3737,.F.);
#5178=ORIENTED_EDGE('',*,*,#3738,.F.);
#5179=ORIENTED_EDGE('',*,*,#3676,.T.);
#5180=ORIENTED_EDGE('',*,*,#3621,.T.);
#5181=ORIENTED_EDGE('',*,*,#3633,.T.);
#5182=ORIENTED_EDGE('',*,*,#3734,.T.);
#5183=ORIENTED_EDGE('',*,*,#3689,.F.);
#5184=ORIENTED_EDGE('',*,*,#3739,.T.);
#5185=ORIENTED_EDGE('',*,*,#3740,.T.);
#5186=ORIENTED_EDGE('',*,*,#3735,.T.);
#5187=ORIENTED_EDGE('',*,*,#3740,.F.);
#5188=ORIENTED_EDGE('',*,*,#3741,.F.);
#5189=ORIENTED_EDGE('',*,*,#3742,.F.);
#5190=ORIENTED_EDGE('',*,*,#3736,.T.);
#5191=ORIENTED_EDGE('',*,*,#3742,.T.);
#5192=ORIENTED_EDGE('',*,*,#3743,.T.);
#5193=ORIENTED_EDGE('',*,*,#3744,.T.);
#5194=ORIENTED_EDGE('',*,*,#3738,.T.);
#5195=ORIENTED_EDGE('',*,*,#3745,.T.);
#5196=ORIENTED_EDGE('',*,*,#3746,.T.);
#5197=ORIENTED_EDGE('',*,*,#3677,.F.);
#5198=ORIENTED_EDGE('',*,*,#3737,.T.);
#5199=ORIENTED_EDGE('',*,*,#3744,.F.);
#5200=ORIENTED_EDGE('',*,*,#3747,.F.);
#5201=ORIENTED_EDGE('',*,*,#3745,.F.);
#5202=ORIENTED_EDGE('',*,*,#3748,.T.);
#5203=ORIENTED_EDGE('',*,*,#3749,.T.);
#5204=ORIENTED_EDGE('',*,*,#3747,.T.);
#5205=ORIENTED_EDGE('',*,*,#3750,.T.);
#5206=ORIENTED_EDGE('',*,*,#3751,.T.);
#5207=ORIENTED_EDGE('',*,*,#3752,.T.);
#5208=ORIENTED_EDGE('',*,*,#3741,.T.);
#5209=ORIENTED_EDGE('',*,*,#3753,.T.);
#5210=ORIENTED_EDGE('',*,*,#3754,.T.);
#5211=ORIENTED_EDGE('',*,*,#3748,.F.);
#5212=ORIENTED_EDGE('',*,*,#3743,.F.);
#5213=ORIENTED_EDGE('',*,*,#3754,.F.);
#5214=ORIENTED_EDGE('',*,*,#3667,.F.);
#5215=ORIENTED_EDGE('',*,*,#3688,.F.);
#5216=ORIENTED_EDGE('',*,*,#3668,.F.);
#5217=ORIENTED_EDGE('',*,*,#3753,.F.);
#5218=ORIENTED_EDGE('',*,*,#3739,.F.);
#5219=ORIENTED_EDGE('',*,*,#3755,.T.);
#5220=ORIENTED_EDGE('',*,*,#3713,.T.);
#5221=ORIENTED_EDGE('',*,*,#3756,.T.);
#5222=ORIENTED_EDGE('',*,*,#3756,.F.);
#5223=ORIENTED_EDGE('',*,*,#3715,.F.);
#5224=ORIENTED_EDGE('',*,*,#3752,.F.);
#5225=ORIENTED_EDGE('',*,*,#3757,.F.);
#5226=ORIENTED_EDGE('',*,*,#3696,.F.);
#5227=ORIENTED_EDGE('',*,*,#3711,.F.);
#5228=ORIENTED_EDGE('',*,*,#3755,.F.);
#5229=ORIENTED_EDGE('',*,*,#3758,.F.);
#5230=ORIENTED_EDGE('',*,*,#3698,.F.);
#5231=ORIENTED_EDGE('',*,*,#3759,.F.);
#5232=ORIENTED_EDGE('',*,*,#3751,.F.);
#5233=ORIENTED_EDGE('',*,*,#3716,.F.);
#5234=ORIENTED_EDGE('',*,*,#3706,.T.);
#5235=ORIENTED_EDGE('',*,*,#3717,.F.);
#5236=ORIENTED_EDGE('',*,*,#3750,.F.);
#5237=ORIENTED_EDGE('',*,*,#3714,.F.);
#5238=ORIENTED_EDGE('',*,*,#3678,.F.);
#5239=ORIENTED_EDGE('',*,*,#3746,.F.);
#5240=ORIENTED_EDGE('',*,*,#3749,.F.);
#5241=ORIENTED_EDGE('',*,*,#3666,.F.);
#5242=ORIENTED_EDGE('',*,*,#3758,.T.);
#5243=ORIENTED_EDGE('',*,*,#3757,.T.);
#5244=ORIENTED_EDGE('',*,*,#3759,.T.);
#5245=ORIENTED_EDGE('',*,*,#3697,.F.);
#5246=ORIENTED_EDGE('',*,*,#3760,.F.);
#5247=ORIENTED_EDGE('',*,*,#3761,.F.);
#5248=ORIENTED_EDGE('',*,*,#3762,.F.);
#5249=ORIENTED_EDGE('',*,*,#3763,.F.);
#5250=ORIENTED_EDGE('',*,*,#3764,.F.);
#5251=ORIENTED_EDGE('',*,*,#3765,.F.);
#5252=ORIENTED_EDGE('',*,*,#3766,.F.);
#5253=ORIENTED_EDGE('',*,*,#3767,.F.);
#5254=ORIENTED_EDGE('',*,*,#3768,.F.);
#5255=ORIENTED_EDGE('',*,*,#3760,.T.);
#5256=ORIENTED_EDGE('',*,*,#3769,.T.);
#5257=ORIENTED_EDGE('',*,*,#3767,.T.);
#5258=ORIENTED_EDGE('',*,*,#3770,.T.);
#5259=ORIENTED_EDGE('',*,*,#3686,.T.);
#5260=ORIENTED_EDGE('',*,*,#3771,.T.);
#5261=ORIENTED_EDGE('',*,*,#3768,.T.);
#5262=ORIENTED_EDGE('',*,*,#3772,.T.);
#5263=ORIENTED_EDGE('',*,*,#3773,.F.);
#5264=ORIENTED_EDGE('',*,*,#3774,.F.);
#5265=ORIENTED_EDGE('',*,*,#3775,.F.);
#5266=ORIENTED_EDGE('',*,*,#3774,.T.);
#5267=ORIENTED_EDGE('',*,*,#3776,.T.);
#5268=ORIENTED_EDGE('',*,*,#3764,.T.);
#5269=ORIENTED_EDGE('',*,*,#3777,.T.);
#5270=ORIENTED_EDGE('',*,*,#3766,.T.);
#5271=ORIENTED_EDGE('',*,*,#3778,.T.);
#5272=ORIENTED_EDGE('',*,*,#3775,.T.);
#5273=ORIENTED_EDGE('',*,*,#3779,.T.);
#5274=ORIENTED_EDGE('',*,*,#3684,.T.);
#5275=ORIENTED_EDGE('',*,*,#3780,.T.);
#5276=ORIENTED_EDGE('',*,*,#3773,.T.);
#5277=ORIENTED_EDGE('',*,*,#3781,.T.);
#5278=ORIENTED_EDGE('',*,*,#3682,.T.);
#5279=ORIENTED_EDGE('',*,*,#3782,.T.);
#5280=ORIENTED_EDGE('',*,*,#3765,.T.);
#5281=ORIENTED_EDGE('',*,*,#3783,.T.);
#5282=ORIENTED_EDGE('',*,*,#3763,.T.);
#5283=ORIENTED_EDGE('',*,*,#3784,.T.);
#5284=ORIENTED_EDGE('',*,*,#3761,.T.);
#5285=ORIENTED_EDGE('',*,*,#3785,.T.);
#5286=ORIENTED_EDGE('',*,*,#3680,.T.);
#5287=ORIENTED_EDGE('',*,*,#3786,.T.);
#5288=ORIENTED_EDGE('',*,*,#3762,.T.);
#5289=ORIENTED_EDGE('',*,*,#3787,.T.);
#5290=ORIENTED_EDGE('',*,*,#3781,.F.);
#5291=ORIENTED_EDGE('',*,*,#3778,.F.);
#5292=ORIENTED_EDGE('',*,*,#3771,.F.);
#5293=ORIENTED_EDGE('',*,*,#3685,.F.);
#5294=ORIENTED_EDGE('',*,*,#3603,.T.);
#5295=ORIENTED_EDGE('',*,*,#3687,.F.);
#5296=ORIENTED_EDGE('',*,*,#3772,.F.);
#5297=ORIENTED_EDGE('',*,*,#3769,.F.);
#5298=ORIENTED_EDGE('',*,*,#3786,.F.);
#5299=ORIENTED_EDGE('',*,*,#3679,.F.);
#5300=ORIENTED_EDGE('',*,*,#3619,.T.);
#5301=ORIENTED_EDGE('',*,*,#3632,.T.);
#5302=ORIENTED_EDGE('',*,*,#3777,.F.);
#5303=ORIENTED_EDGE('',*,*,#3785,.F.);
#5304=ORIENTED_EDGE('',*,*,#3770,.F.);
#5305=ORIENTED_EDGE('',*,*,#3779,.F.);
#5306=ORIENTED_EDGE('',*,*,#3549,.T.);
#5307=ORIENTED_EDGE('',*,*,#3565,.T.);
#5308=ORIENTED_EDGE('',*,*,#3562,.T.);
#5309=ORIENTED_EDGE('',*,*,#3559,.T.);
#5310=ORIENTED_EDGE('',*,*,#3556,.T.);
#5311=ORIENTED_EDGE('',*,*,#3553,.T.);
#5312=ORIENTED_EDGE('',*,*,#3568,.T.);
#5313=ORIENTED_EDGE('',*,*,#3584,.T.);
#5314=ORIENTED_EDGE('',*,*,#3581,.T.);
#5315=ORIENTED_EDGE('',*,*,#3578,.T.);
#5316=ORIENTED_EDGE('',*,*,#3575,.T.);
#5317=ORIENTED_EDGE('',*,*,#3572,.T.);
#5318=ORIENTED_EDGE('',*,*,#3595,.T.);
#5319=ORIENTED_EDGE('',*,*,#3592,.T.);
#5320=ORIENTED_EDGE('',*,*,#3589,.T.);
#5321=ORIENTED_EDGE('',*,*,#3587,.T.);
#5322=ORIENTED_EDGE('',*,*,#3782,.F.);
#5323=ORIENTED_EDGE('',*,*,#3681,.F.);
#5324=ORIENTED_EDGE('',*,*,#3787,.F.);
#5325=ORIENTED_EDGE('',*,*,#3784,.F.);
#5326=ORIENTED_EDGE('',*,*,#3780,.F.);
#5327=ORIENTED_EDGE('',*,*,#3683,.F.);
#5328=ORIENTED_EDGE('',*,*,#3783,.F.);
#5329=ORIENTED_EDGE('',*,*,#3776,.F.);
#6063=CYLINDRICAL_SURFACE('',#6833,0.25);
#6064=CYLINDRICAL_SURFACE('',#6835,0.25);
#6065=CYLINDRICAL_SURFACE('',#6837,0.25);
#6066=CYLINDRICAL_SURFACE('',#6839,0.25);
#6067=CYLINDRICAL_SURFACE('',#6861,0.15);
#6068=CYLINDRICAL_SURFACE('',#6863,0.15);
#6069=CYLINDRICAL_SURFACE('',#6866,0.15);
#6070=CYLINDRICAL_SURFACE('',#6869,0.15);
#6071=CYLINDRICAL_SURFACE('',#6871,0.17);
#6072=CYLINDRICAL_SURFACE('',#6873,0.17);
#6073=CYLINDRICAL_SURFACE('',#6897,0.4);
#6074=CYLINDRICAL_SURFACE('',#6898,0.4);
#6075=CYLINDRICAL_SURFACE('',#6921,0.1);
#6076=CYLINDRICAL_SURFACE('',#6925,0.1);
#6077=CYLINDRICAL_SURFACE('',#6939,0.3);
#6078=CYLINDRICAL_SURFACE('',#6944,0.3);
#6303=ADVANCED_FACE('',(#931),#6063,.F.);
#6304=ADVANCED_FACE('',(#932),#6064,.F.);
#6305=ADVANCED_FACE('',(#933),#6065,.F.);
#6306=ADVANCED_FACE('',(#934),#6066,.F.);
#6307=ADVANCED_FACE('',(#935),#124,.T.);
#6308=ADVANCED_FACE('',(#936),#125,.T.);
#6309=ADVANCED_FACE('',(#937,#616,#617,#618),#717,.F.);
#6310=ADVANCED_FACE('',(#938),#718,.F.);
#6311=ADVANCED_FACE('',(#939),#719,.F.);
#6312=ADVANCED_FACE('',(#940),#720,.F.);
#6313=ADVANCED_FACE('',(#941),#721,.F.);
#6314=ADVANCED_FACE('',(#942),#722,.F.);
#6315=ADVANCED_FACE('',(#943),#723,.F.);
#6316=ADVANCED_FACE('',(#944,#619),#724,.F.);
#6317=ADVANCED_FACE('',(#945),#725,.F.);
#6318=ADVANCED_FACE('',(#946),#726,.F.);
#6319=ADVANCED_FACE('',(#947),#727,.F.);
#6320=ADVANCED_FACE('',(#948),#728,.F.);
#6321=ADVANCED_FACE('',(#949),#729,.F.);
#6322=ADVANCED_FACE('',(#950),#730,.F.);
#6323=ADVANCED_FACE('',(#951,#620),#731,.F.);
#6324=ADVANCED_FACE('',(#952),#6067,.F.);
#6325=ADVANCED_FACE('',(#953),#6068,.F.);
#6326=ADVANCED_FACE('',(#954),#6069,.F.);
#6327=ADVANCED_FACE('',(#955),#6070,.F.);
#6328=ADVANCED_FACE('',(#956),#6071,.F.);
#6329=ADVANCED_FACE('',(#957),#6072,.F.);
#6330=ADVANCED_FACE('',(#958),#732,.F.);
#6331=ADVANCED_FACE('',(#959),#733,.F.);
#6332=ADVANCED_FACE('',(#960),#734,.F.);
#6333=ADVANCED_FACE('',(#961),#735,.F.);
#6334=ADVANCED_FACE('',(#962),#736,.F.);
#6335=ADVANCED_FACE('',(#963),#737,.F.);
#6336=ADVANCED_FACE('',(#964),#738,.F.);
#6337=ADVANCED_FACE('',(#965,#621),#739,.F.);
#6338=ADVANCED_FACE('',(#966,#622),#740,.F.);
#6339=ADVANCED_FACE('',(#967),#741,.F.);
#6340=ADVANCED_FACE('',(#968),#742,.F.);
#6341=ADVANCED_FACE('',(#969),#743,.F.);
#6342=ADVANCED_FACE('',(#970),#744,.F.);
#6343=ADVANCED_FACE('',(#971),#745,.F.);
#6344=ADVANCED_FACE('',(#972),#746,.T.);
#6345=ADVANCED_FACE('',(#973),#747,.T.);
#6346=ADVANCED_FACE('',(#974),#748,.T.);
#6347=ADVANCED_FACE('',(#975),#749,.T.);
#6348=ADVANCED_FACE('',(#976),#750,.T.);
#6349=ADVANCED_FACE('',(#977,#623),#751,.F.);
#6350=ADVANCED_FACE('',(#978),#6073,.T.);
#6351=ADVANCED_FACE('',(#979),#6074,.T.);
#6352=ADVANCED_FACE('',(#980),#752,.T.);
#6353=ADVANCED_FACE('',(#981),#126,.T.);
#6354=ADVANCED_FACE('',(#982),#127,.T.);
#6355=ADVANCED_FACE('',(#983),#128,.T.);
#6356=ADVANCED_FACE('',(#984),#129,.T.);
#6357=ADVANCED_FACE('',(#985),#753,.F.);
#6358=ADVANCED_FACE('',(#986),#130,.T.);
#6359=ADVANCED_FACE('',(#987),#131,.T.);
#6360=ADVANCED_FACE('',(#988),#754,.T.);
#6361=ADVANCED_FACE('',(#989),#132,.T.);
#6362=ADVANCED_FACE('',(#990),#133,.T.);
#6363=ADVANCED_FACE('',(#991),#755,.F.);
#6364=ADVANCED_FACE('',(#992),#134,.T.);
#6365=ADVANCED_FACE('',(#993),#135,.T.);
#6366=ADVANCED_FACE('',(#994),#756,.T.);
#6367=ADVANCED_FACE('',(#995),#136,.T.);
#6368=ADVANCED_FACE('',(#996),#137,.T.);
#6369=ADVANCED_FACE('',(#997,#624,#625,#626),#757,.F.);
#6370=ADVANCED_FACE('',(#998),#138,.T.);
#6371=ADVANCED_FACE('',(#999),#758,.T.);
#6372=ADVANCED_FACE('',(#1000),#139,.T.);
#6373=ADVANCED_FACE('',(#1001),#140,.T.);
#6374=ADVANCED_FACE('',(#1002),#759,.F.);
#6375=ADVANCED_FACE('',(#1003),#141,.T.);
#6376=ADVANCED_FACE('',(#1004),#142,.T.);
#6377=ADVANCED_FACE('',(#1005),#84,.F.);
#6378=ADVANCED_FACE('',(#1006),#85,.F.);
#6379=ADVANCED_FACE('',(#1007),#86,.F.);
#6380=ADVANCED_FACE('',(#1008),#6075,.F.);
#6381=ADVANCED_FACE('',(#1009),#143,.T.);
#6382=ADVANCED_FACE('',(#1010),#87,.F.);
#6383=ADVANCED_FACE('',(#1011),#6076,.F.);
#6384=ADVANCED_FACE('',(#1012),#144,.T.);
#6385=ADVANCED_FACE('',(#1013),#145,.T.);
#6386=ADVANCED_FACE('',(#1014),#146,.T.);
#6387=ADVANCED_FACE('',(#1015),#147,.T.);
#6388=ADVANCED_FACE('',(#1016),#760,.T.);
#6389=ADVANCED_FACE('',(#1017),#88,.T.);
#6390=ADVANCED_FACE('',(#1018),#89,.T.);
#6391=ADVANCED_FACE('',(#1019),#90,.T.);
#6392=ADVANCED_FACE('',(#1020),#6077,.T.);
#6393=ADVANCED_FACE('',(#1021),#148,.F.);
#6394=ADVANCED_FACE('',(#1022),#91,.T.);
#6395=ADVANCED_FACE('',(#1023),#6078,.T.);
#6396=ADVANCED_FACE('',(#1024),#149,.F.);
#6397=ADVANCED_FACE('',(#1025),#150,.F.);
#6398=ADVANCED_FACE('',(#1026),#151,.F.);
#6399=ADVANCED_FACE('',(#1027),#152,.F.);
#6400=ADVANCED_FACE('',(#1028),#153,.F.);
#6401=ADVANCED_FACE('',(#1029),#154,.F.);
#6402=ADVANCED_FACE('',(#1030),#761,.F.);
#6403=ADVANCED_FACE('',(#1031,#627,#628,#629,#630,#631,#632),#762,.T.);
#6404=ADVANCED_FACE('',(#1032),#155,.F.);
#6405=ADVANCED_FACE('',(#1033),#763,.F.);
#6548=CLOSED_SHELL('',(#6303,#6304,#6305,#6306,#6307,#6308,#6309,#6310,
#6311,#6312,#6313,#6314,#6315,#6316,#6317,#6318,#6319,#6320,#6321,#6322,
#6323,#6324,#6325,#6326,#6327,#6328,#6329,#6330,#6331,#6332,#6333,#6334,
#6335,#6336,#6337,#6338,#6339,#6340,#6341,#6342,#6343,#6344,#6345,#6346,
#6347,#6348,#6349,#6350,#6351,#6352,#6353,#6354,#6355,#6356,#6357,#6358,
#6359,#6360,#6361,#6362,#6363,#6364,#6365,#6366,#6367,#6368,#6369,#6370,
#6371,#6372,#6373,#6374,#6375,#6376,#6377,#6378,#6379,#6380,#6381,#6382,
#6383,#6384,#6385,#6386,#6387,#6388,#6389,#6390,#6391,#6392,#6393,#6394,
#6395,#6396,#6397,#6398,#6399,#6400,#6401,#6402,#6403,#6404,#6405));
#6832=AXIS2_PLACEMENT_3D('',#10756,#7653,#7654);
#6833=AXIS2_PLACEMENT_3D('',#10757,#7655,#7656);
#6834=AXIS2_PLACEMENT_3D('',#10784,#7657,#7658);
#6835=AXIS2_PLACEMENT_3D('',#10785,#7659,#7660);
#6836=AXIS2_PLACEMENT_3D('',#10808,#7661,#7662);
#6837=AXIS2_PLACEMENT_3D('',#10809,#7663,#7664);
#6838=AXIS2_PLACEMENT_3D('',#10832,#7665,#7666);
#6839=AXIS2_PLACEMENT_3D('',#10833,#7667,#7668);
#6840=AXIS2_PLACEMENT_3D('',#10860,#7669,#7670);
#6841=AXIS2_PLACEMENT_3D('',#11045,#7671,#7672);
#6842=AXIS2_PLACEMENT_3D('',#11059,#7675,#7676);
#6843=AXIS2_PLACEMENT_3D('',#11061,#7677,#7678);
#6844=AXIS2_PLACEMENT_3D('',#11063,#7679,#7680);
#6845=AXIS2_PLACEMENT_3D('',#11064,#7681,#7682);
#6846=AXIS2_PLACEMENT_3D('',#11073,#7687,#7688);
#6847=AXIS2_PLACEMENT_3D('',#11079,#7692,#7693);
#6848=AXIS2_PLACEMENT_3D('',#11085,#7697,#7698);
#6849=AXIS2_PLACEMENT_3D('',#11091,#7702,#7703);
#6850=AXIS2_PLACEMENT_3D('',#11097,#7707,#7708);
#6851=AXIS2_PLACEMENT_3D('',#11100,#7711,#7712);
#6852=AXIS2_PLACEMENT_3D('',#11102,#7713,#7714);
#6853=AXIS2_PLACEMENT_3D('',#11103,#7715,#7716);
#6854=AXIS2_PLACEMENT_3D('',#11112,#7721,#7722);
#6855=AXIS2_PLACEMENT_3D('',#11118,#7726,#7727);
#6856=AXIS2_PLACEMENT_3D('',#11124,#7731,#7732);
#6857=AXIS2_PLACEMENT_3D('',#11130,#7736,#7737);
#6858=AXIS2_PLACEMENT_3D('',#11136,#7741,#7742);
#6859=AXIS2_PLACEMENT_3D('',#11139,#7745,#7746);
#6860=AXIS2_PLACEMENT_3D('',#11141,#7747,#7748);
#6861=AXIS2_PLACEMENT_3D('',#11142,#7749,#7750);
#6862=AXIS2_PLACEMENT_3D('',#11144,#7751,#7752);
#6863=AXIS2_PLACEMENT_3D('',#11146,#7754,#7755);
#6864=AXIS2_PLACEMENT_3D('',#11148,#7756,#7757);
#6865=AXIS2_PLACEMENT_3D('',#11151,#7759,#7760);
#6866=AXIS2_PLACEMENT_3D('',#11152,#7761,#7762);
#6867=AXIS2_PLACEMENT_3D('',#11154,#7763,#7764);
#6868=AXIS2_PLACEMENT_3D('',#11157,#7766,#7767);
#6869=AXIS2_PLACEMENT_3D('',#11158,#7768,#7769);
#6870=AXIS2_PLACEMENT_3D('',#11160,#7770,#7771);
#6871=AXIS2_PLACEMENT_3D('',#11162,#7773,#7774);
#6872=AXIS2_PLACEMENT_3D('',#11165,#7776,#7777);
#6873=AXIS2_PLACEMENT_3D('',#11166,#7778,#7779);
#6874=AXIS2_PLACEMENT_3D('',#11169,#7781,#7782);
#6875=AXIS2_PLACEMENT_3D('',#11170,#7783,#7784);
#6876=AXIS2_PLACEMENT_3D('',#11179,#7789,#7790);
#6877=AXIS2_PLACEMENT_3D('',#11188,#7795,#7796);
#6878=AXIS2_PLACEMENT_3D('',#11197,#7801,#7802);
#6879=AXIS2_PLACEMENT_3D('',#11206,#7807,#7808);
#6880=AXIS2_PLACEMENT_3D('',#11215,#7813,#7814);
#6881=AXIS2_PLACEMENT_3D('',#11224,#7819,#7820);
#6882=AXIS2_PLACEMENT_3D('',#11233,#7825,#7826);
#6883=AXIS2_PLACEMENT_3D('',#11235,#7827,#7828);
#6884=AXIS2_PLACEMENT_3D('',#11236,#7829,#7830);
#6885=AXIS2_PLACEMENT_3D('',#11238,#7831,#7832);
#6886=AXIS2_PLACEMENT_3D('',#11239,#7833,#7834);
#6887=AXIS2_PLACEMENT_3D('',#11242,#7837,#7838);
#6888=AXIS2_PLACEMENT_3D('',#11245,#7841,#7842);
#6889=AXIS2_PLACEMENT_3D('',#11248,#7845,#7846);
#6890=AXIS2_PLACEMENT_3D('',#11254,#7850,#7851);
#6891=AXIS2_PLACEMENT_3D('',#11260,#7855,#7856);
#6892=AXIS2_PLACEMENT_3D('',#11305,#7858,#7859);
#6893=AXIS2_PLACEMENT_3D('',#11351,#7862,#7863);
#6894=AXIS2_PLACEMENT_3D('',#11429,#7867,#7868);
#6895=AXIS2_PLACEMENT_3D('',#11477,#7872,#7873);
#6896=AXIS2_PLACEMENT_3D('',#11493,#7877,#7878);
#6897=AXIS2_PLACEMENT_3D('',#11814,#7890,#7891);
#6898=AXIS2_PLACEMENT_3D('',#11816,#7893,#7894);
#6899=AXIS2_PLACEMENT_3D('',#11818,#7895,#7896);
#6900=AXIS2_PLACEMENT_3D('',#11820,#7898,#7899);
#6901=AXIS2_PLACEMENT_3D('',#11984,#7901,#7902);
#6902=AXIS2_PLACEMENT_3D('',#11985,#7903,#7904);
#6903=AXIS2_PLACEMENT_3D('',#12033,#7906,#7907);
#6904=AXIS2_PLACEMENT_3D('',#12151,#7909,#7910);
#6905=AXIS2_PLACEMENT_3D('',#12196,#7911,#7912);
#6906=AXIS2_PLACEMENT_3D('',#12288,#7914,#7915);
#6907=AXIS2_PLACEMENT_3D('',#12305,#7916,#7917);
#6908=AXIS2_PLACEMENT_3D('',#12425,#7919,#7920);
#6909=AXIS2_PLACEMENT_3D('',#12430,#7921,#7922);
#6910=AXIS2_PLACEMENT_3D('',#12482,#7924,#7925);
#6911=AXIS2_PLACEMENT_3D('',#12483,#7926,#7927);
#6912=AXIS2_PLACEMENT_3D('',#12484,#7928,#7929);
#6913=AXIS2_PLACEMENT_3D('',#12485,#7930,#7931);
#6914=AXIS2_PLACEMENT_3D('',#12486,#7932,#7933);
#6915=AXIS2_PLACEMENT_3D('',#12487,#7934,#7935);
#6916=AXIS2_PLACEMENT_3D('',#12489,#7936,#7937);
#6917=AXIS2_PLACEMENT_3D('',#12490,#7938,#7939);
#6918=AXIS2_PLACEMENT_3D('',#12491,#7940,#7941);
#6919=AXIS2_PLACEMENT_3D('',#12492,#7942,#7943);
#6920=AXIS2_PLACEMENT_3D('',#12493,#7944,#7945);
#6921=AXIS2_PLACEMENT_3D('',#12494,#7946,#7947);
#6922=AXIS2_PLACEMENT_3D('',#12515,#7948,#7949);
#6923=AXIS2_PLACEMENT_3D('',#12517,#7950,#7951);
#6924=AXIS2_PLACEMENT_3D('',#12518,#7952,#7953);
#6925=AXIS2_PLACEMENT_3D('',#12519,#7954,#7955);
#6926=AXIS2_PLACEMENT_3D('',#12609,#7957,#7958);
#6927=AXIS2_PLACEMENT_3D('',#12610,#7959,#7960);
#6928=AXIS2_PLACEMENT_3D('',#12613,#7961,#7962);
#6929=AXIS2_PLACEMENT_3D('',#12615,#7963,#7964);
#6930=AXIS2_PLACEMENT_3D('',#12616,#7965,#7966);
#6931=AXIS2_PLACEMENT_3D('',#12617,#7967,#7968);
#6932=AXIS2_PLACEMENT_3D('',#12620,#7969,#7970);
#6933=AXIS2_PLACEMENT_3D('',#12622,#7971,#7972);
#6934=AXIS2_PLACEMENT_3D('',#12623,#7973,#7974);
#6935=AXIS2_PLACEMENT_3D('',#12624,#7975,#7976);
#6936=AXIS2_PLACEMENT_3D('',#12627,#7977,#7978);
#6937=AXIS2_PLACEMENT_3D('',#12629,#7979,#7980);
#6938=AXIS2_PLACEMENT_3D('',#12630,#7981,#7982);
#6939=AXIS2_PLACEMENT_3D('',#12631,#7983,#7984);
#6940=AXIS2_PLACEMENT_3D('',#12662,#7987,#7988);
#6941=AXIS2_PLACEMENT_3D('',#12665,#7989,#7990);
#6942=AXIS2_PLACEMENT_3D('',#12667,#7991,#7992);
#6943=AXIS2_PLACEMENT_3D('',#12668,#7993,#7994);
#6944=AXIS2_PLACEMENT_3D('',#12669,#7995,#7996);
#6945=AXIS2_PLACEMENT_3D('',#12842,#7999,#8000);
#6946=AXIS2_PLACEMENT_3D('',#12843,#8001,#8002);
#6947=AXIS2_PLACEMENT_3D('',#12860,#8003,#8004);
#7653=DIRECTION('axis',(0.,0.,1.));
#7654=DIRECTION('refdir',(1.,0.,0.));
#7655=DIRECTION('center_axis',(0.,0.,-1.));
#7656=DIRECTION('ref_axis',(1.,0.,0.));
#7657=DIRECTION('center_axis',(0.,0.,1.));
#7658=DIRECTION('ref_axis',(1.,0.,0.));
#7659=DIRECTION('center_axis',(0.,0.,-1.));
#7660=DIRECTION('ref_axis',(1.,0.,0.));
#7661=DIRECTION('center_axis',(0.,0.,1.));
#7662=DIRECTION('ref_axis',(1.,0.,0.));
#7663=DIRECTION('center_axis',(0.,0.,-1.));
#7664=DIRECTION('ref_axis',(1.,0.,0.));
#7665=DIRECTION('center_axis',(0.,0.,1.));
#7666=DIRECTION('ref_axis',(1.,0.,0.));
#7667=DIRECTION('center_axis',(0.,0.,-1.));
#7668=DIRECTION('ref_axis',(1.,0.,0.));
#7669=DIRECTION('center_axis',(0.,0.,1.));
#7670=DIRECTION('ref_axis',(1.,0.,0.));
#7671=DIRECTION('center_axis',(4.10828654779316E-33,-1.13946463231163E-19,
1.));
#7672=DIRECTION('ref_axis',(1.,0.,-4.10828654779316E-33));
#7673=DIRECTION('',(0.,1.,1.13946463231163E-19));
#7674=DIRECTION('',(0.,-1.,-1.13946463231163E-19));
#7675=DIRECTION('center_axis',(4.10828654779316E-33,-1.13946463231163E-19,
1.));
#7676=DIRECTION('ref_axis',(1.,0.,0.));
#7677=DIRECTION('center_axis',(4.10828654779316E-33,-1.13946463231163E-19,
1.));
#7678=DIRECTION('ref_axis',(1.,0.,0.));
#7679=DIRECTION('center_axis',(4.10828654779316E-33,-1.13946463231163E-19,
1.));
#7680=DIRECTION('ref_axis',(1.,0.,0.));
#7681=DIRECTION('center_axis',(0.86602540378444,0.499999999999998,0.));
#7682=DIRECTION('ref_axis',(0.499999999999998,-0.86602540378444,0.));
#7683=DIRECTION('',(0.499999999999998,-0.86602540378444,-9.86805318295791E-20));
#7684=DIRECTION('',(0.,0.,-1.));
#7685=DIRECTION('',(0.499999999999998,-0.86602540378444,0.));
#7686=DIRECTION('',(0.,0.,-1.));
#7687=DIRECTION('center_axis',(1.60246890531964E-16,1.,0.));
#7688=DIRECTION('ref_axis',(1.,-1.60246890531964E-16,0.));
#7689=DIRECTION('',(1.,-1.60246890531964E-16,-4.12654611421307E-33));
#7690=DIRECTION('',(0.,0.,-1.));
#7691=DIRECTION('',(1.,-1.60246890531964E-16,0.));
#7692=DIRECTION('center_axis',(-0.86602540378444,0.499999999999998,0.));
#7693=DIRECTION('ref_axis',(0.499999999999998,0.86602540378444,0.));
#7694=DIRECTION('',(0.499999999999998,0.86602540378444,9.86805318295749E-20));
#7695=DIRECTION('',(0.,0.,-1.));
#7696=DIRECTION('',(0.499999999999998,0.86602540378444,0.));
#7697=DIRECTION('center_axis',(-0.86602540378444,-0.499999999999998,0.));
#7698=DIRECTION('ref_axis',(-0.499999999999998,0.86602540378444,0.));
#7699=DIRECTION('',(-0.499999999999998,0.86602540378444,9.86805318295791E-20));
#7700=DIRECTION('',(0.,0.,-1.));
#7701=DIRECTION('',(-0.499999999999998,0.86602540378444,0.));
#7702=DIRECTION('center_axis',(-1.60246890531964E-16,-1.,0.));
#7703=DIRECTION('ref_axis',(-1.,1.60246890531964E-16,0.));
#7704=DIRECTION('',(-1.,1.60246890531964E-16,4.12654611421307E-33));
#7705=DIRECTION('',(0.,0.,-1.));
#7706=DIRECTION('',(-1.,1.60246890531964E-16,0.));
#7707=DIRECTION('center_axis',(0.86602540378444,-0.499999999999998,0.));
#7708=DIRECTION('ref_axis',(-0.499999999999998,-0.86602540378444,0.));
#7709=DIRECTION('',(-0.499999999999998,-0.86602540378444,-9.86805318295749E-20));
#7710=DIRECTION('',(-0.499999999999998,-0.86602540378444,0.));
#7711=DIRECTION('center_axis',(0.,0.,-1.));
#7712=DIRECTION('ref_axis',(-1.,0.,0.));
#7713=DIRECTION('center_axis',(0.,0.,1.));
#7714=DIRECTION('ref_axis',(1.,0.,0.));
#7715=DIRECTION('center_axis',(0.866025403784439,0.5,0.));
#7716=DIRECTION('ref_axis',(0.5,-0.866025403784439,0.));
#7717=DIRECTION('',(0.5,-0.866025403784439,-9.86805318295789E-20));
#7718=DIRECTION('',(0.,0.,-1.));
#7719=DIRECTION('',(0.5,-0.866025403784439,0.));
#7720=DIRECTION('',(0.,0.,-1.));
#7721=DIRECTION('center_axis',(1.60246890531964E-16,1.,0.));
#7722=DIRECTION('ref_axis',(1.,-1.60246890531964E-16,0.));
#7723=DIRECTION('',(1.,-1.60246890531964E-16,-4.12654611421307E-33));
#7724=DIRECTION('',(0.,0.,-1.));
#7725=DIRECTION('',(1.,-1.60246890531964E-16,0.));
#7726=DIRECTION('center_axis',(-0.866025403784438,0.5,0.));
#7727=DIRECTION('ref_axis',(0.5,0.866025403784438,0.));
#7728=DIRECTION('',(0.5,0.866025403784438,9.86805318295748E-20));
#7729=DIRECTION('',(0.,0.,-1.));
#7730=DIRECTION('',(0.5,0.866025403784438,0.));
#7731=DIRECTION('center_axis',(-0.866025403784439,-0.499999999999999,0.));
#7732=DIRECTION('ref_axis',(-0.499999999999999,0.866025403784439,0.));
#7733=DIRECTION('',(-0.499999999999999,0.866025403784439,9.8680531829579E-20));
#7734=DIRECTION('',(0.,0.,-1.));
#7735=DIRECTION('',(-0.499999999999999,0.866025403784439,0.));
#7736=DIRECTION('center_axis',(-1.60246890531964E-16,-1.,0.));
#7737=DIRECTION('ref_axis',(-1.,1.60246890531964E-16,0.));
#7738=DIRECTION('',(-1.,1.60246890531964E-16,4.12654611421307E-33));
#7739=DIRECTION('',(0.,0.,-1.));
#7740=DIRECTION('',(-1.,1.60246890531964E-16,0.));
#7741=DIRECTION('center_axis',(0.866025403784439,-0.5,0.));
#7742=DIRECTION('ref_axis',(-0.5,-0.866025403784439,0.));
#7743=DIRECTION('',(-0.5,-0.866025403784439,-9.86805318295748E-20));
#7744=DIRECTION('',(-0.5,-0.866025403784439,0.));
#7745=DIRECTION('center_axis',(0.,0.,-1.));
#7746=DIRECTION('ref_axis',(-1.,0.,0.));
#7747=DIRECTION('center_axis',(0.,0.,1.));
#7748=DIRECTION('ref_axis',(1.,0.,0.));
#7749=DIRECTION('center_axis',(0.,0.,-1.));
#7750=DIRECTION('ref_axis',(1.,0.,0.));
#7751=DIRECTION('center_axis',(-4.10828654779316E-33,1.13946463231163E-19,
-1.));
#7752=DIRECTION('ref_axis',(1.,0.,0.));
#7753=DIRECTION('',(0.,0.,-1.));
#7754=DIRECTION('center_axis',(0.,0.,-1.));
#7755=DIRECTION('ref_axis',(1.,0.,0.));
#7756=DIRECTION('center_axis',(-4.10828654779316E-33,1.13946463231163E-19,
-1.));
#7757=DIRECTION('ref_axis',(1.,0.,0.));
#7758=DIRECTION('',(0.,0.,-1.));
#7759=DIRECTION('center_axis',(4.10828654779316E-33,-1.13946463231163E-19,
1.));
#7760=DIRECTION('ref_axis',(1.,0.,0.));
#7761=DIRECTION('center_axis',(0.,0.,-1.));
#7762=DIRECTION('ref_axis',(1.,0.,0.));
#7763=DIRECTION('center_axis',(-4.10828654779316E-33,1.13946463231163E-19,
-1.));
#7764=DIRECTION('ref_axis',(1.,0.,0.));
#7765=DIRECTION('',(0.,0.,-1.));
#7766=DIRECTION('center_axis',(4.10828654779316E-33,-1.13946463231163E-19,
1.));
#7767=DIRECTION('ref_axis',(1.,0.,0.));
#7768=DIRECTION('center_axis',(0.,0.,-1.));
#7769=DIRECTION('ref_axis',(1.,0.,0.));
#7770=DIRECTION('center_axis',(-4.10828654779316E-33,1.13946463231163E-19,
-1.));
#7771=DIRECTION('ref_axis',(1.,0.,0.));
#7772=DIRECTION('',(0.,0.,-1.));
#7773=DIRECTION('center_axis',(0.,0.,-1.));
#7774=DIRECTION('ref_axis',(1.,0.,0.));
#7775=DIRECTION('',(0.,0.,-1.));
#7776=DIRECTION('center_axis',(0.,0.,1.));
#7777=DIRECTION('ref_axis',(1.,0.,0.));
#7778=DIRECTION('center_axis',(0.,0.,-1.));
#7779=DIRECTION('ref_axis',(1.,0.,0.));
#7780=DIRECTION('',(0.,0.,-1.));
#7781=DIRECTION('center_axis',(0.,0.,1.));
#7782=DIRECTION('ref_axis',(1.,0.,0.));
#7783=DIRECTION('center_axis',(0.,-1.,0.));
#7784=DIRECTION('ref_axis',(-1.,0.,0.));
#7785=DIRECTION('',(0.0523359562429438,0.,0.998629534754574));
#7786=DIRECTION('',(1.,0.,0.));
#7787=DIRECTION('',(-0.0523359562429438,0.,-0.998629534754574));
#7788=DIRECTION('',(1.,0.,0.));
#7789=DIRECTION('center_axis',(0.,-1.,0.));
#7790=DIRECTION('ref_axis',(-1.,0.,0.));
#7791=DIRECTION('',(0.,0.,-1.));
#7792=DIRECTION('',(1.,0.,0.));
#7793=DIRECTION('',(0.,0.,1.));
#7794=DIRECTION('',(1.,0.,0.));
#7795=DIRECTION('center_axis',(0.,-1.,0.));
#7796=DIRECTION('ref_axis',(-1.,0.,0.));
#7797=DIRECTION('',(0.,0.,-1.));
#7798=DIRECTION('',(1.,0.,0.));
#7799=DIRECTION('',(0.,0.,1.));
#7800=DIRECTION('',(1.,0.,0.));
#7801=DIRECTION('center_axis',(0.,-1.,0.));
#7802=DIRECTION('ref_axis',(-1.,0.,0.));
#7803=DIRECTION('',(0.,0.,-1.));
#7804=DIRECTION('',(1.,0.,0.));
#7805=DIRECTION('',(0.,0.,1.));
#7806=DIRECTION('',(1.,0.,0.));
#7807=DIRECTION('center_axis',(0.,1.,0.));
#7808=DIRECTION('ref_axis',(1.,0.,0.));
#7809=DIRECTION('',(-0.0523359562429438,0.,-0.998629534754574));
#7810=DIRECTION('',(-1.,0.,0.));
#7811=DIRECTION('',(0.0523359562429438,0.,0.998629534754574));
#7812=DIRECTION('',(-1.,0.,0.));
#7813=DIRECTION('center_axis',(0.,1.,0.));
#7814=DIRECTION('ref_axis',(1.,0.,0.));
#7815=DIRECTION('',(0.,0.,1.));
#7816=DIRECTION('',(-1.,0.,0.));
#7817=DIRECTION('',(0.,0.,-1.));
#7818=DIRECTION('',(-1.,0.,0.));
#7819=DIRECTION('center_axis',(0.,1.,0.));
#7820=DIRECTION('ref_axis',(1.,0.,0.));
#7821=DIRECTION('',(0.,0.,1.));
#7822=DIRECTION('',(-1.,0.,0.));
#7823=DIRECTION('',(0.,0.,-1.));
#7824=DIRECTION('',(-1.,0.,0.));
#7825=DIRECTION('center_axis',(0.,0.,1.));
#7826=DIRECTION('ref_axis',(1.,0.,0.));
#7827=DIRECTION('center_axis',(0.,0.,1.));
#7828=DIRECTION('ref_axis',(1.,0.,0.));
#7829=DIRECTION('center_axis',(0.,0.,1.));
#7830=DIRECTION('ref_axis',(1.,0.,0.));
#7831=DIRECTION('center_axis',(0.,0.,1.));
#7832=DIRECTION('ref_axis',(1.,0.,0.));
#7833=DIRECTION('center_axis',(0.,0.,1.));
#7834=DIRECTION('ref_axis',(1.,0.,0.));
#7835=DIRECTION('',(0.,1.,0.));
#7836=DIRECTION('',(0.,-1.,0.));
#7837=DIRECTION('center_axis',(0.,0.,1.));
#7838=DIRECTION('ref_axis',(1.,0.,0.));
#7839=DIRECTION('',(0.,-1.,0.));
#7840=DIRECTION('',(0.,1.,0.));
#7841=DIRECTION('center_axis',(0.,0.,1.));
#7842=DIRECTION('ref_axis',(1.,0.,0.));
#7843=DIRECTION('',(0.,-1.,0.));
#7844=DIRECTION('',(0.,1.,0.));
#7845=DIRECTION('center_axis',(0.,0.,1.));
#7846=DIRECTION('ref_axis',(1.,0.,0.));
#7847=DIRECTION('',(0.,-1.,0.));
#7848=DIRECTION('',(-1.,0.,0.));
#7849=DIRECTION('',(0.,1.,0.));
#7850=DIRECTION('center_axis',(0.,1.,0.));
#7851=DIRECTION('ref_axis',(1.,0.,0.));
#7852=DIRECTION('',(0.,0.,1.));
#7853=DIRECTION('',(-1.,0.,0.));
#7854=DIRECTION('',(0.,0.,-1.));
#7855=DIRECTION('center_axis',(-1.,0.,0.));
#7856=DIRECTION('ref_axis',(0.,-1.,0.));
#7857=DIRECTION('',(0.,-1.,0.));
#7858=DIRECTION('center_axis',(1.,0.,0.));
#7859=DIRECTION('ref_axis',(0.,1.,0.));
#7860=DIRECTION('',(0.,1.,0.));
#7861=DIRECTION('',(0.,1.,0.));
#7862=DIRECTION('center_axis',(1.,0.,0.));
#7863=DIRECTION('ref_axis',(0.,1.,0.));
#7864=DIRECTION('',(0.,1.,0.));
#7865=DIRECTION('',(0.,1.,1.13946463231163E-19));
#7866=DIRECTION('',(0.,1.,0.));
#7867=DIRECTION('center_axis',(1.,0.,0.));
#7868=DIRECTION('ref_axis',(0.,1.,0.));
#7869=DIRECTION('',(0.,1.,0.));
#7870=DIRECTION('',(0.,1.,1.13946463231163E-19));
#7871=DIRECTION('',(0.,1.,0.));
#7872=DIRECTION('center_axis',(0.998629534754574,0.,-0.0523359562429438));
#7873=DIRECTION('ref_axis',(-0.0523359562429438,0.,-0.998629534754574));
#7874=DIRECTION('',(0.,-1.,0.));
#7875=DIRECTION('',(-5.97168109510197E-21,-1.,-1.13946463231163E-19));
#7876=DIRECTION('',(0.,-1.,0.));
#7877=DIRECTION('center_axis',(0.,0.,1.));
#7878=DIRECTION('ref_axis',(1.,0.,0.));
#7879=DIRECTION('',(0.,-1.,0.));
#7880=DIRECTION('',(0.,-1.,0.));
#7881=DIRECTION('',(0.,-1.,0.));
#7882=DIRECTION('',(0.,1.,0.));
#7883=DIRECTION('',(0.,-1.,0.));
#7884=DIRECTION('',(0.,1.,0.));
#7885=DIRECTION('',(0.,-1.,0.));
#7886=DIRECTION('',(0.,-1.,0.));
#7887=DIRECTION('',(0.,-1.,0.));
#7888=DIRECTION('',(0.,1.,0.));
#7889=DIRECTION('',(0.,1.,0.));
#7890=DIRECTION('center_axis',(0.,0.,1.));
#7891=DIRECTION('ref_axis',(1.,0.,0.));
#7892=DIRECTION('',(0.,0.,-1.));
#7893=DIRECTION('center_axis',(0.,0.,1.));
#7894=DIRECTION('ref_axis',(1.,0.,0.));
#7895=DIRECTION('center_axis',(4.10828654779316E-33,-1.13946463231163E-19,
1.));
#7896=DIRECTION('ref_axis',(1.,0.,0.));
#7897=DIRECTION('',(0.,0.,-1.));
#7898=DIRECTION('center_axis',(1.,0.,0.));
#7899=DIRECTION('ref_axis',(0.,1.,0.));
#7900=DIRECTION('',(0.,1.,1.13946463231163E-19));
#7901=DIRECTION('center_axis',(0.99852593895705,0.0542765992849681,9.38276897523041E-9));
#7902=DIRECTION('ref_axis',(0.0541946171271057,-0.99701772369063,0.0549418066794405));
#7903=DIRECTION('center_axis',(4.10828654779316E-33,-1.13946463231163E-19,
1.));
#7904=DIRECTION('ref_axis',(1.,0.,-4.10828654779316E-33));
#7905=DIRECTION('',(5.97168109510217E-21,-1.,-1.13946463231163E-19));
#7906=DIRECTION('center_axis',(-1.,0.,0.));
#7907=DIRECTION('ref_axis',(0.,-1.,0.));
#7908=DIRECTION('',(0.,-1.,-1.13946463231163E-19));
#7909=DIRECTION('center_axis',(4.10828654779316E-33,-1.13946463231163E-19,
1.));
#7910=DIRECTION('ref_axis',(1.,0.,-4.10828654779316E-33));
#7911=DIRECTION('center_axis',(-1.,0.,0.));
#7912=DIRECTION('ref_axis',(0.,-1.,0.));
#7913=DIRECTION('',(0.,-1.,-1.13946463231163E-19));
#7914=DIRECTION('center_axis',(4.10828654779316E-33,-1.13946463231163E-19,
1.));
#7915=DIRECTION('ref_axis',(1.,0.,-4.10828654779316E-33));
#7916=DIRECTION('center_axis',(-1.,0.,0.));
#7917=DIRECTION('ref_axis',(0.,-1.,0.));
#7918=DIRECTION('',(0.,-1.,-1.13946463231163E-19));
#7919=DIRECTION('center_axis',(-0.996961060527779,0.0779015005717205,0.));
#7920=DIRECTION('ref_axis',(0.,0.,1.));
#7921=DIRECTION('center_axis',(4.10828654779316E-33,-1.13946463231163E-19,
1.));
#7922=DIRECTION('ref_axis',(1.,0.,-4.10828654779316E-33));
#7923=DIRECTION('',(5.97168109510197E-21,1.,1.13946463231163E-19));
#7924=DIRECTION('center_axis',(-0.996961060527779,-0.0779015005717276,-4.485055189269E-15));
#7925=DIRECTION('ref_axis',(-0.0777791112471086,0.995394757055134,0.0560329142626144));
#7926=DIRECTION('center_axis',(-0.377317868652411,-0.840644185582845,0.388521015186253));
#7927=DIRECTION('ref_axis',(-0.58566693710526,0.541587807512093,0.603056287203763));
#7928=DIRECTION('center_axis',(7.41164423166535E-16,1.,0.));
#7929=DIRECTION('ref_axis',(0.,0.,1.));
#7930=DIRECTION('center_axis',(0.0522650005536027,-0.0520548592672972,0.997275619547472));
#7931=DIRECTION('ref_axis',(-0.998629534754574,7.40148683083438E-16,0.0523359562429445));
#7932=DIRECTION('center_axis',(0.376559988603802,-0.837471124372148,0.396036224133039));
#7933=DIRECTION('ref_axis',(0.577069986161316,0.546481578685729,0.606916893181374));
#7934=DIRECTION('center_axis',(0.998525938475037,-0.0542766081525538,0.));
#7935=DIRECTION('ref_axis',(0.,0.,1.));
#7936=DIRECTION('center_axis',(-0.0522648366634829,-0.0521149007022807,
0.997272492337641));
#7937=DIRECTION('ref_axis',(0.0541946171271058,0.99701772369063,0.0549418066794413));
#7938=DIRECTION('center_axis',(5.32220538281047E-11,1.,-1.01553728389566E-9));
#7939=DIRECTION('ref_axis',(0.998629534754574,0.,0.0523359562429456));
#7940=DIRECTION('center_axis',(0.37731786865241,-0.840644185582843,-0.388521015186259));
#7941=DIRECTION('ref_axis',(-0.585666937105255,-0.541587807512096,0.603056287203765));
#7942=DIRECTION('center_axis',(0.0522650005536027,0.0520548592672965,0.997275619547472));
#7943=DIRECTION('ref_axis',(-0.0777791112471059,-0.995394757055134,0.0560329142626137));
#7944=DIRECTION('center_axis',(0.,-1.,0.));
#7945=DIRECTION('ref_axis',(-0.998629534754574,0.,0.0523359562429439));
#7946=DIRECTION('center_axis',(5.97168109510197E-21,1.,1.13946463231163E-19));
#7947=DIRECTION('ref_axis',(-0.688354575693753,0.,0.725374371012288));
#7948=DIRECTION('center_axis',(-0.376559987018669,-0.837471124206646,-0.396036225990193));
#7949=DIRECTION('ref_axis',(0.577069983350267,-0.54648157893936,0.606916895625808));
#7950=DIRECTION('center_axis',(-0.0522648366634817,0.0521149007022785,0.997272492337641));
#7951=DIRECTION('ref_axis',(0.998629534754574,0.,0.052335956242946));
#7952=DIRECTION('center_axis',(1.01693095242295E-9,-1.,0.));
#7953=DIRECTION('ref_axis',(0.,0.,1.));
#7954=DIRECTION('center_axis',(5.97168109510217E-21,-1.,-1.13946463231163E-19));
#7955=DIRECTION('ref_axis',(0.688354575693753,0.,0.725374371012289));
#7956=DIRECTION('',(-5.97168109510217E-21,1.,1.13946463231163E-19));
#7957=DIRECTION('center_axis',(-0.998629534754574,0.,-0.0523359562429455));
#7958=DIRECTION('ref_axis',(-0.0523359562429455,0.,0.998629534754574));
#7959=DIRECTION('center_axis',(-0.377317868652411,-0.840644185582845,0.388521015186254));
#7960=DIRECTION('ref_axis',(-0.585666937105261,0.541587807512092,0.603056287203763));
#7961=DIRECTION('center_axis',(7.41164423166535E-16,1.,0.));
#7962=DIRECTION('ref_axis',(0.,0.,1.));
#7963=DIRECTION('center_axis',(-0.996961060527779,-0.0779015005717276,-4.485055189269E-15));
#7964=DIRECTION('ref_axis',(-0.0777791112471086,0.995394757055134,0.0560329142626144));
#7965=DIRECTION('center_axis',(0.0522650005536027,-0.0520548592672972,0.997275619547472));
#7966=DIRECTION('ref_axis',(-0.998629534754574,7.40148683083438E-16,0.0523359562429445));
#7967=DIRECTION('center_axis',(0.376559988603802,-0.837471124372148,0.396036224133039));
#7968=DIRECTION('ref_axis',(0.577069986161311,0.546481578685732,0.606916893181376));
#7969=DIRECTION('center_axis',(0.998525938475037,-0.0542766081525538,0.));
#7970=DIRECTION('ref_axis',(0.,0.,1.));
#7971=DIRECTION('center_axis',(5.32220538281047E-11,1.,-1.01553728389566E-9));
#7972=DIRECTION('ref_axis',(0.998629534754574,0.,0.0523359562429456));
#7973=DIRECTION('center_axis',(-0.0522648366634829,-0.0521149007022807,
0.997272492337641));
#7974=DIRECTION('ref_axis',(0.0541946171271058,0.99701772369063,0.0549418066794413));
#7975=DIRECTION('center_axis',(0.37731786865241,-0.840644185582843,-0.388521015186259));
#7976=DIRECTION('ref_axis',(-0.585666937105255,-0.541587807512095,0.603056287203766));
#7977=DIRECTION('center_axis',(-0.996961060527779,0.0779015005717205,0.));
#7978=DIRECTION('ref_axis',(0.,0.,1.));
#7979=DIRECTION('center_axis',(0.,-1.,0.));
#7980=DIRECTION('ref_axis',(-0.998629534754574,0.,0.0523359562429439));
#7981=DIRECTION('center_axis',(0.0522650005536027,0.0520548592672965,0.997275619547472));
#7982=DIRECTION('ref_axis',(-0.0777791112471059,-0.995394757055134,0.0560329142626137));
#7983=DIRECTION('center_axis',(5.97168109510197E-21,1.,1.13946463231163E-19));
#7984=DIRECTION('ref_axis',(-0.688354575693753,0.,0.725374371012289));
#7985=DIRECTION('',(-5.97168109510197E-21,-1.,-1.13946463231163E-19));
#7986=DIRECTION('',(5.97168109510197E-21,1.,1.13946463231163E-19));
#7987=DIRECTION('center_axis',(-0.376559987018669,-0.837471124206646,-0.396036225990194));
#7988=DIRECTION('ref_axis',(0.577069983350267,-0.546481578939359,0.606916895625808));
#7989=DIRECTION('center_axis',(-0.0522648366634817,0.0521149007022785,0.997272492337641));
#7990=DIRECTION('ref_axis',(0.998629534754574,0.,0.052335956242946));
#7991=DIRECTION('center_axis',(1.01693095242295E-9,-1.,0.));
#7992=DIRECTION('ref_axis',(0.,0.,1.));
#7993=DIRECTION('center_axis',(0.99852593895705,0.0542765992849681,9.38276897523041E-9));
#7994=DIRECTION('ref_axis',(0.0541946171271057,-0.99701772369063,0.0549418066794405));
#7995=DIRECTION('center_axis',(5.97168109510217E-21,-1.,-1.13946463231163E-19));
#7996=DIRECTION('ref_axis',(0.688354575693753,0.,0.725374371012289));
#7997=DIRECTION('',(-5.97168109510217E-21,1.,1.13946463231163E-19));
#7998=DIRECTION('',(5.97168109510217E-21,-1.,-1.13946463231163E-19));
#7999=DIRECTION('center_axis',(0.998629534754574,0.,-0.0523359562429438));
#8000=DIRECTION('ref_axis',(-0.0523359562429438,0.,-0.998629534754574));
#8001=DIRECTION('center_axis',(4.10828654779316E-33,-1.13946463231163E-19,
1.));
#8002=DIRECTION('ref_axis',(1.,0.,-4.10828654779316E-33));
#8003=DIRECTION('center_axis',(-0.998629534754574,0.,-0.0523359562429455));
#8004=DIRECTION('ref_axis',(-0.0523359562429455,0.,0.998629534754574));
#10756=CARTESIAN_POINT('',(0.,0.,0.));
#10757=CARTESIAN_POINT('Origin',(8.1,-1.,0.7));
#10758=CARTESIAN_POINT('',(7.94916965151797,-1.19937453693185,0.7));
#10759=CARTESIAN_POINT('',(8.26514540988519,-1.18768855477586,0.7));
#10760=CARTESIAN_POINT('Ctrl Pts',(7.94916965151797,-1.19937453693185,0.7));
#10761=CARTESIAN_POINT('Ctrl Pts',(7.97160858810976,-1.21634998764782,0.7));
#10762=CARTESIAN_POINT('Ctrl Pts',(7.99739856866269,-1.22989011121344,0.69528529300377));
#10763=CARTESIAN_POINT('Ctrl Pts',(8.03944443766207,-1.24298414277179,0.688517705185315));
#10764=CARTESIAN_POINT('Ctrl Pts',(8.05362924383607,-1.24609346022897,0.686388676887586));
#10765=CARTESIAN_POINT('Ctrl Pts',(8.075506183533,-1.24890990228851,0.684139035126277));
#10766=CARTESIAN_POINT('Ctrl Pts',(8.08297567221474,-1.24953307703463,0.683546226354886));
#10767=CARTESIAN_POINT('Ctrl Pts',(8.0940066533036,-1.24995288972095,0.68299521602547));
#10768=CARTESIAN_POINT('Ctrl Pts',(8.09752287926269,-1.25001251279495,0.68286729538075));
#10769=CARTESIAN_POINT('Ctrl Pts',(8.10293413375911,-1.249989933108,0.682747340264197));
#10770=CARTESIAN_POINT('Ctrl Pts',(8.10482478940148,-1.24996059450444,0.682719828470948));
#10771=CARTESIAN_POINT('Ctrl Pts',(8.10828546792054,-1.24986760009171,0.682696100760705));
#10772=CARTESIAN_POINT('Ctrl Pts',(8.10985478687837,-1.24981062779486,0.682695370268813));
#10773=CARTESIAN_POINT('Ctrl Pts',(8.11326464342549,-1.24965465239671,0.682715595753076));
#10774=CARTESIAN_POINT('Ctrl Pts',(8.11510409202247,-1.2495501177419,0.682740330911594));
#10775=CARTESIAN_POINT('Ctrl Pts',(8.12014207260669,-1.24920790966494,0.682845651127781));
#10776=CARTESIAN_POINT('Ctrl Pts',(8.12333423895876,-1.24892926854386,0.682953992816581));
#10777=CARTESIAN_POINT('Ctrl Pts',(8.139194120874,-1.2472372768871,0.683691668462565));
#10778=CARTESIAN_POINT('Ctrl Pts',(8.15164141295685,-1.2449338270761,0.684918799511701));
#10779=CARTESIAN_POINT('Ctrl Pts',(8.19196937649467,-1.23428099896052,0.690212518998986));
#10780=CARTESIAN_POINT('Ctrl Pts',(8.21811504697062,-1.22213176592155,0.695755006185672));
#10781=CARTESIAN_POINT('Ctrl Pts',(8.24962874265135,-1.20052913769617,0.699397421419897));
#10782=CARTESIAN_POINT('Ctrl Pts',(8.25758631484639,-1.19433973204149,0.7));
#10783=CARTESIAN_POINT('Ctrl Pts',(8.26514540988519,-1.18768855477586,0.7));
#10784=CARTESIAN_POINT('Origin',(8.1,-1.,0.7));
#10785=CARTESIAN_POINT('Origin',(2.7,1.,0.7));
#10786=CARTESIAN_POINT('',(2.8076286513348,1.22564590451442,0.7));
#10787=CARTESIAN_POINT('',(2.57739843082973,1.21787348447435,0.7));
#10788=CARTESIAN_POINT('Ctrl Pts',(2.80762864495888,1.22564590575571,0.7));
#10789=CARTESIAN_POINT('Ctrl Pts',(2.78743249310418,1.23527907171202,0.7));
#10790=CARTESIAN_POINT('Ctrl Pts',(2.76507271635938,1.24261561512899,0.698430289974852));
#10791=CARTESIAN_POINT('Ctrl Pts',(2.73219941643314,1.24807722603274,0.696876198609429));
#10792=CARTESIAN_POINT('Ctrl Pts',(2.72335305886828,1.24906618730719,0.696525251810408));
#10793=CARTESIAN_POINT('Ctrl Pts',(2.71018695034311,1.24982905432238,0.696188910804419));
#10794=CARTESIAN_POINT('Ctrl Pts',(2.70590779780308,1.24996687586326,0.696107915309552));
#10795=CARTESIAN_POINT('Ctrl Pts',(2.69921702211412,1.25001037316246,0.696030339680738));
#10796=CARTESIAN_POINT('Ctrl Pts',(2.69680890442544,1.24999123464332,0.696012302673685));
#10797=CARTESIAN_POINT('Ctrl Pts',(2.69234597975348,1.24989125947742,0.695997601992606));
#10798=CARTESIAN_POINT('Ctrl Pts',(2.69029169500035,1.24981988388707,0.69599819279703));
#10799=CARTESIAN_POINT('Ctrl Pts',(2.6857660481318,1.24960673159635,0.696015705561832));
#10800=CARTESIAN_POINT('Ctrl Pts',(2.68329599580702,1.24945360531346,0.696035938105249));
#10801=CARTESIAN_POINT('Ctrl Pts',(2.67625328071593,1.24891193026541,0.696123377063474));
#10802=CARTESIAN_POINT('Ctrl Pts',(2.67169109188753,1.24843439216159,0.696216059649547));
#10803=CARTESIAN_POINT('Ctrl Pts',(2.64765560351845,1.24524789167778,0.696873729305584));
#10804=CARTESIAN_POINT('Ctrl Pts',(2.62857598726268,1.24037162800668,0.698048768812303));
#10805=CARTESIAN_POINT('Ctrl Pts',(2.59902076831046,1.22902239593109,0.699541037747764));
#10806=CARTESIAN_POINT('Ctrl Pts',(2.58799157881597,1.22383445108162,0.7));
#10807=CARTESIAN_POINT('Ctrl Pts',(2.57739843082979,1.21787348447436,0.7));
#10808=CARTESIAN_POINT('Origin',(2.7,1.,0.7));
#10809=CARTESIAN_POINT('Origin',(2.7,-1.,0.7));
#10810=CARTESIAN_POINT('',(2.57739843082979,-1.21787348447436,0.7));
#10811=CARTESIAN_POINT('',(2.80762864495888,-1.22564590575571,0.7));
#10812=CARTESIAN_POINT('Ctrl Pts',(2.57739843082979,-1.21787348447436,0.7));
#10813=CARTESIAN_POINT('Ctrl Pts',(2.59689796709118,-1.22884624579732,0.7));
#10814=CARTESIAN_POINT('Ctrl Pts',(2.61871070177046,-1.23767364961455,0.698430520021629));
#10815=CARTESIAN_POINT('Ctrl Pts',(2.6511387549791,-1.24533993869645,0.696876447160353));
#10816=CARTESIAN_POINT('Ctrl Pts',(2.65989793055836,-1.24692336726652,0.696525471319567));
#10817=CARTESIAN_POINT('Ctrl Pts',(2.67298219502323,-1.24857266139659,0.696189053183015));
#10818=CARTESIAN_POINT('Ctrl Pts',(2.67724223626036,-1.24899884484677,0.696108027479433));
#10819=CARTESIAN_POINT('Ctrl Pts',(2.68391475503581,-1.24949361628703,0.696030400846995));
#10820=CARTESIAN_POINT('Ctrl Pts',(2.68631866330158,-1.24963697932539,0.69601234479389));
#10821=CARTESIAN_POINT('Ctrl Pts',(2.69077815115796,-1.24983831390468,0.695997608323079));
#10822=CARTESIAN_POINT('Ctrl Pts',(2.69283257145917,-1.24990568929416,0.695998182544699));
#10823=CARTESIAN_POINT('Ctrl Pts',(2.69736230434386,-1.24999833696454,0.696015659042177));
#10824=CARTESIAN_POINT('Ctrl Pts',(2.69983707579759,-1.25001219669429,0.696035872086962));
#10825=CARTESIAN_POINT('Ctrl Pts',(2.70690037992806,-1.24994687665095,0.696123257636812));
#10826=CARTESIAN_POINT('Ctrl Pts',(2.71148446565418,-1.24977820005943,0.696215908504701));
#10827=CARTESIAN_POINT('Ctrl Pts',(2.73568105999059,-1.24822038288304,0.696873447340259));
#10828=CARTESIAN_POINT('Ctrl Pts',(2.75504695022812,-1.24464213141243,0.698048515307351));
#10829=CARTESIAN_POINT('Ctrl Pts',(2.78530198112344,-1.2353118289445,0.699540950501024));
#10830=CARTESIAN_POINT('Ctrl Pts',(2.79665680001786,-1.23087925931356,0.7));
#10831=CARTESIAN_POINT('Ctrl Pts',(2.80762864495888,-1.22564590575571,0.7));
#10832=CARTESIAN_POINT('Origin',(2.7,-1.,0.7));
#10833=CARTESIAN_POINT('Origin',(8.1,1.,0.7));
#10834=CARTESIAN_POINT('',(8.26514540988519,1.18768855477586,0.7));
#10835=CARTESIAN_POINT('',(7.94916965249954,1.19937453719419,0.7));
#10836=CARTESIAN_POINT('Ctrl Pts',(8.26514540988519,1.18768855477586,0.7));
#10837=CARTESIAN_POINT('Ctrl Pts',(8.24402114884725,1.20627559516199,0.7));
#10838=CARTESIAN_POINT('Ctrl Pts',(8.21930102059268,1.22168408824046,0.695284768760077));
#10839=CARTESIAN_POINT('Ctrl Pts',(8.17833936508797,1.23784683595578,0.688517484674842));
#10840=CARTESIAN_POINT('Ctrl Pts',(8.16442627443898,1.24199461640617,0.686388979601913));
#10841=CARTESIAN_POINT('Ctrl Pts',(8.14282164862934,1.24641910835203,0.684139556285851));
#10842=CARTESIAN_POINT('Ctrl Pts',(8.13541969045672,1.24759243465272,0.683546718614312));
#10843=CARTESIAN_POINT('Ctrl Pts',(8.12445132655127,1.24882623938238,0.682995554842566));
#10844=CARTESIAN_POINT('Ctrl Pts',(8.12094947916695,1.24914555886372,0.68286756899844));
#10845=CARTESIAN_POINT('Ctrl Pts',(8.11555178799172,1.24952297970176,0.682747494033431));
#10846=CARTESIAN_POINT('Ctrl Pts',(8.11366421100955,1.24963346420394,0.682719937279798));
#10847=CARTESIAN_POINT('Ctrl Pts',(8.11020620287515,1.24979651712922,0.682696124556263));
#10848=CARTESIAN_POINT('Ctrl Pts',(8.10863696767328,1.24985569708818,0.682695355189016));
#10849=CARTESIAN_POINT('Ctrl Pts',(8.10522484403353,1.249952190393,0.682715496638402));
#10850=CARTESIAN_POINT('Ctrl Pts',(8.10338263267786,1.24998390529834,0.682740187713169));
#10851=CARTESIAN_POINT('Ctrl Pts',(8.09833277498968,1.25001501472208,0.682845394223802));
#10852=CARTESIAN_POINT('Ctrl Pts',(8.09512844909059,1.24997307323179,0.682953673497893));
#10853=CARTESIAN_POINT('Ctrl Pts',(8.07918314804204,1.24945780552822,0.683691186949858));
#10854=CARTESIAN_POINT('Ctrl Pts',(8.06659630270856,1.24808001426183,0.684918585227095));
#10855=CARTESIAN_POINT('Ctrl Pts',(8.02558960427868,1.24043495378573,0.69021260546313));
#10856=CARTESIAN_POINT('Ctrl Pts',(7.9986188553413,1.2302509517108,0.695754623970086));
#10857=CARTESIAN_POINT('Ctrl Pts',(7.96559475436581,1.21103543221342,0.69939729083119));
#10858=CARTESIAN_POINT('Ctrl Pts',(7.95720051358587,1.20545002552208,0.7));
#10859=CARTESIAN_POINT('Ctrl Pts',(7.94916965151797,1.19937453693185,0.7));
#10860=CARTESIAN_POINT('Origin',(8.1,1.,0.7));
#10861=CARTESIAN_POINT('Ctrl Pts',(1.1,1.14549341399196,0.7));
#10862=CARTESIAN_POINT('Ctrl Pts',(1.89984199608574,1.1957170361627,0.7));
#10863=CARTESIAN_POINT('Ctrl Pts',(2.70080437300401,1.2273695200909,0.7));
#10864=CARTESIAN_POINT('Ctrl Pts',(3.50204003610941,1.24374118183538,0.7));
#10865=CARTESIAN_POINT('Ctrl Pts',(1.09819048660397,1.17431102498992,0.7));
#10866=CARTESIAN_POINT('Ctrl Pts',(1.89847848223077,1.22458382597074,0.70000077422621));
#10867=CARTESIAN_POINT('Ctrl Pts',(2.69984520196781,1.25626413437997,0.699999727319846));
#10868=CARTESIAN_POINT('Ctrl Pts',(3.50144932661635,1.27265074030048,0.700000000000001));
#10869=CARTESIAN_POINT('Ctrl Pts',(1.09505363188407,1.22426736091617,0.676703190608825));
#10870=CARTESIAN_POINT('Ctrl Pts',(1.89610976425884,1.27462253270773,0.67666760713801));
#10871=CARTESIAN_POINT('Ctrl Pts',(2.69818680938115,1.3063522351595,0.67664530655333));
#10872=CARTESIAN_POINT('Ctrl Pts',(3.50042536655637,1.322763754511,0.676632802377821));
#10873=CARTESIAN_POINT('Ctrl Pts',(1.09381704710221,1.24396073223232,0.627109609335854));
#10874=CARTESIAN_POINT('Ctrl Pts',(1.89518106151152,1.29430885982199,0.62701751976321));
#10875=CARTESIAN_POINT('Ctrl Pts',(2.69753328610131,1.32603127467068,0.626959208652505));
#10876=CARTESIAN_POINT('Ctrl Pts',(3.50002334924346,1.34243864233338,0.626926882269943));
#10877=CARTESIAN_POINT('Ctrl Pts',(1.09374258853658,1.24514653057163,0.605486452199395));
#10878=CARTESIAN_POINT('Ctrl Pts',(1.89512529323683,1.29547288309274,0.605377720397184));
#10879=CARTESIAN_POINT('Ctrl Pts',(2.69749615303001,1.32718177535833,0.605308474776761));
#10880=CARTESIAN_POINT('Ctrl Pts',(3.5,1.34358136363184,0.605270327458635));
#10881=CARTESIAN_POINT('',(1.1,1.14549341399195,0.7));
#10882=CARTESIAN_POINT('Ctrl Pts',(1.1,1.14549341399196,0.7));
#10883=CARTESIAN_POINT('Ctrl Pts',(1.59210562457523,1.17639367564078,0.7));
#10884=CARTESIAN_POINT('Ctrl Pts',(2.08463535466703,1.20026407570248,0.7));
#10885=CARTESIAN_POINT('Ctrl Pts',(2.57739190516306,1.2178709162388,0.7));
#10886=CARTESIAN_POINT('',(1.1,1.24553911298206,0.605485603995113));
#10887=CARTESIAN_POINT('Ctrl Pts',(1.1,1.14549341399196,0.7));
#10888=CARTESIAN_POINT('Ctrl Pts',(1.1,1.15341616150799,0.7));
#10889=CARTESIAN_POINT('Ctrl Pts',(1.1000012416168,1.16127613060545,0.699006361583129));
#10890=CARTESIAN_POINT('Ctrl Pts',(1.10000231308998,1.16893252943985,0.697119293189023));
#10891=CARTESIAN_POINT('Ctrl Pts',(1.10000291357081,1.17322337016277,0.696061732044743));
#10892=CARTESIAN_POINT('Ctrl Pts',(1.10000345673767,1.17745032641463,0.694722535963768));
#10893=CARTESIAN_POINT('Ctrl Pts',(1.10000379529503,1.18158693416151,0.693112479763539));
#10894=CARTESIAN_POINT('Ctrl Pts',(1.1000044034764,1.18901789868739,0.690220189452084));
#10895=CARTESIAN_POINT('Ctrl Pts',(1.1000042334852,1.19607766167095,0.686488065947256));
#10896=CARTESIAN_POINT('Ctrl Pts',(1.10000339376692,1.2026196529327,0.681996646156542));
#10897=CARTESIAN_POINT('Ctrl Pts',(1.10000293249552,1.20621327895058,0.67952943359521));
#10898=CARTESIAN_POINT('Ctrl Pts',(1.10000228571683,1.20965039763183,0.676832226278619));
#10899=CARTESIAN_POINT('Ctrl Pts',(1.10000171524363,1.21290279159005,0.673912896410569));
#10900=CARTESIAN_POINT('Ctrl Pts',(1.10000115816795,1.2160788033717,0.671062126739188));
#10901=CARTESIAN_POINT('Ctrl Pts',(1.10000066850715,1.2190594221245,0.668016750164662));
#10902=CARTESIAN_POINT('Ctrl Pts',(1.10000067525152,1.22182202639256,0.664788091882127));
#10903=CARTESIAN_POINT('Ctrl Pts',(1.10000068775799,1.22694487635592,0.658801012170571));
#10904=CARTESIAN_POINT('Ctrl Pts',(1.10000222199399,1.23132099043293,0.652185071179834));
#10905=CARTESIAN_POINT('Ctrl Pts',(1.10000276904041,1.23488987417606,0.64510534613808));
#10906=CARTESIAN_POINT('Ctrl Pts',(1.10000282439334,1.23525099193115,0.644388983656765));
#10907=CARTESIAN_POINT('Ctrl Pts',(1.10000287212626,1.23560380546488,0.64366785367332));
#10908=CARTESIAN_POINT('Ctrl Pts',(1.10000291138002,1.23594822450451,0.642942116631622));
#10909=CARTESIAN_POINT('Ctrl Pts',(1.10000329911404,1.23935026814133,0.635773555081239));
#10910=CARTESIAN_POINT('Ctrl Pts',(1.10000258010782,1.24189771450306,0.628240464257889));
#10911=CARTESIAN_POINT('Ctrl Pts',(1.10000149084855,1.24353681278199,0.620511076118615));
#10912=CARTESIAN_POINT('Ctrl Pts',(1.10000079446814,1.24458471384188,0.615569557890241));
#10913=CARTESIAN_POINT('Ctrl Pts',(1.10000000111128,1.24526049271905,0.610547146027233));
#10914=CARTESIAN_POINT('Ctrl Pts',(1.09999999916631,1.24553911263843,0.605485603997432));
#10915=CARTESIAN_POINT('',(3.5,1.34358136363184,0.605270327458635));
#10916=CARTESIAN_POINT('Ctrl Pts',(3.5,1.34358136363184,0.605270327458635));
#10917=CARTESIAN_POINT('Ctrl Pts',(2.6995848679345,1.32722445934619,0.605308375488923));
#10918=CARTESIAN_POINT('Ctrl Pts',(1.89930203168261,1.29563783986497,0.605377360150118));
#10919=CARTESIAN_POINT('Ctrl Pts',(1.09999999916631,1.24553911263843,0.605485603997431));
#10920=CARTESIAN_POINT('',(3.5,1.24369946473792,0.7));
#10921=CARTESIAN_POINT('Ctrl Pts',(3.5,1.34358136363184,0.605270327458635));
#10922=CARTESIAN_POINT('Ctrl Pts',(3.5,1.34316359984937,0.613184373088104));
#10923=CARTESIAN_POINT('Ctrl Pts',(3.50000057901142,1.34177887744868,0.621008021569537));
#10924=CARTESIAN_POINT('Ctrl Pts',(3.50000082863025,1.33951086762262,0.628580534231506));
#10925=CARTESIAN_POINT('Ctrl Pts',(3.50000096811,1.33824356956914,0.632811834486987));
#10926=CARTESIAN_POINT('Ctrl Pts',(3.50000102536574,1.33669948631919,0.636964759527324));
#10927=CARTESIAN_POINT('Ctrl Pts',(3.50000098105742,1.334886463945,0.641009258704104));
#10928=CARTESIAN_POINT('Ctrl Pts',(3.50000090179773,1.3316432906201,0.648244145614236));
#10929=CARTESIAN_POINT('Ctrl Pts',(3.50000044940971,1.3275777080273,0.655054131048541));
#10930=CARTESIAN_POINT('Ctrl Pts',(3.50000027423476,1.32275302640998,0.661275670751788));
#10931=CARTESIAN_POINT('Ctrl Pts',(3.50000024156065,1.32185311357394,0.66243612938574));
#10932=CARTESIAN_POINT('Ctrl Pts',(3.50000022115524,1.32092666334894,0.663576045687695));
#10933=CARTESIAN_POINT('Ctrl Pts',(3.50000022069074,1.31997391848392,0.664694242102532));
#10934=CARTESIAN_POINT('Ctrl Pts',(3.50000021976176,1.31806844339147,0.666930617752677));
#10935=CARTESIAN_POINT('Ctrl Pts',(3.50000029790302,1.31605782519,0.669080165434128));
#10936=CARTESIAN_POINT('Ctrl Pts',(3.50000040488465,1.31394946763378,0.671139079687271));
#10937=CARTESIAN_POINT('Ctrl Pts',(3.50000069329649,1.3082655455861,0.6766897075128));
#10938=CARTESIAN_POINT('Ctrl Pts',(3.5000011432336,1.30193818666762,0.681521899278667));
#10939=CARTESIAN_POINT('Ctrl Pts',(3.50000129797765,1.29513115062548,0.68558123547136));
#10940=CARTESIAN_POINT('Ctrl Pts',(3.50000139624096,1.2908086457691,0.688158936000333));
#10941=CARTESIAN_POINT('Ctrl Pts',(3.50000139493488,1.28629176508013,0.690424313967808));
#10942=CARTESIAN_POINT('Ctrl Pts',(3.50000129141552,1.28161680488022,0.692354162840695));
#10943=CARTESIAN_POINT('Ctrl Pts',(3.50000112941005,1.27430059661786,0.695374333209024));
#10944=CARTESIAN_POINT('Ctrl Pts',(3.5000007162179,1.26668229982361,0.697540280949125));
#10945=CARTESIAN_POINT('Ctrl Pts',(3.50000038344698,1.25890895215876,0.698782355543395));
#10946=CARTESIAN_POINT('Ctrl Pts',(3.50000016866387,1.25389173534334,0.699584038140014));
#10947=CARTESIAN_POINT('Ctrl Pts',(3.4999999993056,1.24880933504677,0.69999999987784));
#10948=CARTESIAN_POINT('Ctrl Pts',(3.49999999991873,1.24369946470729,0.7));
#10949=CARTESIAN_POINT('Ctrl Pts',(2.80762377174497,1.22564400643366,0.7));
#10950=CARTESIAN_POINT('Ctrl Pts',(3.03837960601223,1.23298334400942,0.7));
#10951=CARTESIAN_POINT('Ctrl Pts',(3.26917843294065,1.23897560812206,0.7));
#10952=CARTESIAN_POINT('Ctrl Pts',(3.49999999991873,1.24369946470729,0.7));
#10953=CARTESIAN_POINT('Ctrl Pts',(7.29709043526678,1.22049830417059,0.7));
#10954=CARTESIAN_POINT('Ctrl Pts',(8.19846709497879,1.19422430779862,0.7));
#10955=CARTESIAN_POINT('Ctrl Pts',(9.09944331332256,1.15544418981837,0.7));
#10956=CARTESIAN_POINT('Ctrl Pts',(10.,1.10900986674273,0.7));
#10957=CARTESIAN_POINT('Ctrl Pts',(7.29793284700474,1.24939875264889,0.7));
#10958=CARTESIAN_POINT('Ctrl Pts',(8.19957769811722,1.22310890030201,0.699999704549177));
#10959=CARTESIAN_POINT('Ctrl Pts',(9.10076698492607,1.18430758604571,0.700000491839571));
#10960=CARTESIAN_POINT('Ctrl Pts',(10.0014871213396,1.13785139984992,0.7));
#10961=CARTESIAN_POINT('Ctrl Pts',(7.29939288958794,1.29948813715084,0.676630595533454));
#10962=CARTESIAN_POINT('Ctrl Pts',(8.20149954052228,1.27317186922949,0.676644146017132));
#10963=CARTESIAN_POINT('Ctrl Pts',(9.10306300621911,1.23433322993607,0.676664155483857));
#10964=CARTESIAN_POINT('Ctrl Pts',(10.0040646682326,1.18784086746588,0.676686753673613));
#10965=CARTESIAN_POINT('Ctrl Pts',(7.29996660609513,1.31917051289423,0.626939603849942));
#10966=CARTESIAN_POINT('Ctrl Pts',(8.20225661204673,1.29285896783792,0.626974637782525));
#10967=CARTESIAN_POINT('Ctrl Pts',(9.10396596140606,1.25402923300358,0.627026849623412));
#10968=CARTESIAN_POINT('Ctrl Pts',(10.0050807923581,1.20754778500352,0.627085325222079));
#10969=CARTESIAN_POINT('Ctrl Pts',(7.29999999953093,1.32031613471704,0.605285370449856));
#10970=CARTESIAN_POINT('Ctrl Pts',(8.20230020786565,1.29401302889245,0.605326714446839));
#10971=CARTESIAN_POINT('Ctrl Pts',(9.10401978846669,1.25519559703033,0.605388684776982));
#10972=CARTESIAN_POINT('Ctrl Pts',(10.0051416645797,1.20872835322339,0.605457722909465));
#10973=CARTESIAN_POINT('',(7.29999999989017,1.22041345054104,0.7));
#10974=CARTESIAN_POINT('Ctrl Pts',(7.29999999978094,1.22041345055303,0.7));
#10975=CARTESIAN_POINT('Ctrl Pts',(7.51641201913776,1.21409884615949,0.7));
#10976=CARTESIAN_POINT('Ctrl Pts',(7.73280095443524,1.20706364503479,0.7));
#10977=CARTESIAN_POINT('Ctrl Pts',(7.94916654146952,1.19937499621344,0.7));
#10978=CARTESIAN_POINT('',(7.29999999953133,1.3203161347307,0.605285370449834));
#10979=CARTESIAN_POINT('Ctrl Pts',(7.29999999989087,1.22041345054982,0.7));
#10980=CARTESIAN_POINT('Ctrl Pts',(7.30000000079355,1.22832360919786,0.699999999740221));
#10981=CARTESIAN_POINT('Ctrl Pts',(7.29999941101664,1.23617007614594,0.699006006469939));
#10982=CARTESIAN_POINT('Ctrl Pts',(7.29999889581476,1.24381267896118,0.697118889344366));
#10983=CARTESIAN_POINT('Ctrl Pts',(7.29999860583198,1.24811433880851,0.696056720321257));
#10984=CARTESIAN_POINT('Ctrl Pts',(7.29999834128398,1.25235147078274,0.694710570513598));
#10985=CARTESIAN_POINT('Ctrl Pts',(7.29999817264931,1.25649739217805,0.693091458416622));
#10986=CARTESIAN_POINT('Ctrl Pts',(7.29999787070862,1.26392067210813,0.690192435210923));
#10987=CARTESIAN_POINT('Ctrl Pts',(7.29999793286912,1.27097116792553,0.686452948287278));
#10988=CARTESIAN_POINT('Ctrl Pts',(7.2999983123982,1.27750284616821,0.681954753865011));
#10989=CARTESIAN_POINT('Ctrl Pts',(7.2999985213788,1.28109939299731,0.679477906983553));
#10990=CARTESIAN_POINT('Ctrl Pts',(7.29999881895966,1.28453837241868,0.676770138671336));
#10991=CARTESIAN_POINT('Ctrl Pts',(7.29999908362886,1.28779148632494,0.673839551409954));
#10992=CARTESIAN_POINT('Ctrl Pts',(7.29999934163235,1.29096267037196,0.670982771155867));
#10993=CARTESIAN_POINT('Ctrl Pts',(7.29999957112158,1.2939379836903,0.667931525418885));
#10994=CARTESIAN_POINT('Ctrl Pts',(7.29999957127586,1.29669488996436,0.664697318929259));
#10995=CARTESIAN_POINT('Ctrl Pts',(7.29999957156178,1.30180432468448,0.658703293276094));
#10996=CARTESIAN_POINT('Ctrl Pts',(7.29999886995656,1.30616650855536,0.652082235935803));
#10997=CARTESIAN_POINT('Ctrl Pts',(7.29999863193158,1.30972187224872,0.644999691185358));
#10998=CARTESIAN_POINT('Ctrl Pts',(7.29999860759325,1.31008541227461,0.644275492840527));
#10999=CARTESIAN_POINT('Ctrl Pts',(7.29999858692673,1.31044047656777,0.643546449710686));
#11000=CARTESIAN_POINT('Ctrl Pts',(7.29999857034625,1.31078697300061,0.642812727646596));
#11001=CARTESIAN_POINT('Ctrl Pts',(7.29999840819729,1.31417553742296,0.635637287305567));
#11002=CARTESIAN_POINT('Ctrl Pts',(7.29999876577208,1.31670951795567,0.628098908385918));
#11003=CARTESIAN_POINT('Ctrl Pts',(7.29999928780719,1.3183355664444,0.620365998324013));
#11004=CARTESIAN_POINT('Ctrl Pts',(7.29999962266353,1.3193785856694,0.615405768714856));
#11005=CARTESIAN_POINT('Ctrl Pts',(7.3,1.32004717656055,0.610364828659741));
#11006=CARTESIAN_POINT('Ctrl Pts',(7.3,1.32031613470337,0.605285370449877));
#11007=CARTESIAN_POINT('',(10.,1.20899340483173,0.605457329065657));
#11008=CARTESIAN_POINT('Ctrl Pts',(9.99999999968202,1.20899340489109,0.605457329065633));
#11009=CARTESIAN_POINT('Ctrl Pts',(9.10058974048747,1.25534320916473,0.605388449123016));
#11010=CARTESIAN_POINT('Ctrl Pts',(8.20058408060299,1.29406305600824,0.605326635812744));
#11011=CARTESIAN_POINT('Ctrl Pts',(7.29999999953093,1.32031613471704,0.605285370449856));
#11012=CARTESIAN_POINT('',(9.99999999523418,1.1090098672342,0.7));
#11013=CARTESIAN_POINT('Ctrl Pts',(9.99999999968202,1.20899340489109,0.605457329065633));
#11014=CARTESIAN_POINT('Ctrl Pts',(9.99999999887489,1.20856043137698,0.613368813757176));
#11015=CARTESIAN_POINT('Ctrl Pts',(9.99999852309337,1.20715974444566,0.621187403383205));
#11016=CARTESIAN_POINT('Ctrl Pts',(9.99999786661901,1.20487567413208,0.628752957409046));
#11017=CARTESIAN_POINT('Ctrl Pts',(9.9999975031266,1.20361097553651,0.63294203403));
#11018=CARTESIAN_POINT('Ctrl Pts',(9.99999733971606,1.20207445367248,0.63705356322819));
#11019=CARTESIAN_POINT('Ctrl Pts',(9.99999742766416,1.20027388348257,0.64105842070465));
#11020=CARTESIAN_POINT('Ctrl Pts',(9.9999975865154,1.19702170610966,0.6482919664668));
#11021=CARTESIAN_POINT('Ctrl Pts',(9.99999868569093,1.19294650045069,0.655099368158521));
#11022=CARTESIAN_POINT('Ctrl Pts',(9.9999991134218,1.18811276085989,0.661317774786376));
#11023=CARTESIAN_POINT('Ctrl Pts',(9.99999919410111,1.18720101282252,0.662490701033652));
#11024=CARTESIAN_POINT('Ctrl Pts',(9.99999924414009,1.18626214680169,0.663642601192937));
#11025=CARTESIAN_POINT('Ctrl Pts',(9.99999924372355,1.18529642131707,0.664772262763739));
#11026=CARTESIAN_POINT('Ctrl Pts',(9.99999924291654,1.18342543943696,0.666960851926287));
#11027=CARTESIAN_POINT('Ctrl Pts',(9.99999905429896,1.18145367213587,0.669066014649603));
#11028=CARTESIAN_POINT('Ctrl Pts',(9.99999879621773,1.17938809187152,0.671084194359814));
#11029=CARTESIAN_POINT('Ctrl Pts',(9.99999808597787,1.17370361260899,0.676638227242868));
#11030=CARTESIAN_POINT('Ctrl Pts',(9.9999969699445,1.16737553754052,0.681473799108647));
#11031=CARTESIAN_POINT('Ctrl Pts',(9.99999660204079,1.16056788011185,0.685537070165577));
#11032=CARTESIAN_POINT('Ctrl Pts',(9.99999636768906,1.15623145667386,0.688125341392612));
#11033=CARTESIAN_POINT('Ctrl Pts',(9.99999638726733,1.15169947441128,0.690399565850749));
#11034=CARTESIAN_POINT('Ctrl Pts',(9.99999666360534,1.14700857532255,0.692336497939236));
#11035=CARTESIAN_POINT('Ctrl Pts',(9.99999709503399,1.13968497812548,0.695360504669253));
#11036=CARTESIAN_POINT('Ctrl Pts',(9.99999815490668,1.13205884654683,0.697530003145419));
#11037=CARTESIAN_POINT('Ctrl Pts',(9.99999900983214,1.12427739544825,0.698775573347137));
#11038=CARTESIAN_POINT('Ctrl Pts',(9.99999956314479,1.11924119569193,0.699581713521624));
#11039=CARTESIAN_POINT('Ctrl Pts',(10.,1.11413933950174,0.7));
#11040=CARTESIAN_POINT('Ctrl Pts',(10.,1.10900986674273,0.7));
#11041=CARTESIAN_POINT('Ctrl Pts',(8.26514054272776,1.18768929227839,0.7));
#11042=CARTESIAN_POINT('Ctrl Pts',(8.84359655063997,1.16547286645366,0.7));
#11043=CARTESIAN_POINT('Ctrl Pts',(9.42188471826001,1.13881853081542,0.7));
#11044=CARTESIAN_POINT('Ctrl Pts',(9.99999999522154,1.10900986698912,0.7));
#11045=CARTESIAN_POINT('Origin',(5.4,-8.11656130105013E-18,0.7));
#11046=CARTESIAN_POINT('',(7.3,-1.22041345053557,0.7));
#11047=CARTESIAN_POINT('Ctrl Pts',(7.94916654049851,-1.19937499624794,0.7));
#11048=CARTESIAN_POINT('Ctrl Pts',(7.73280095382446,-1.20706364505454,0.7));
#11049=CARTESIAN_POINT('Ctrl Pts',(7.51641201888728,-1.21409884616656,0.7));
#11050=CARTESIAN_POINT('Ctrl Pts',(7.29999999989085,-1.22041345054982,0.7));
#11051=CARTESIAN_POINT('',(7.3,-0.712777777777778,0.7));
#11052=CARTESIAN_POINT('',(10.,-1.10900986674244,0.7));
#11053=CARTESIAN_POINT('',(10.,0.653773457742722,0.7));
#11054=CARTESIAN_POINT('Ctrl Pts',(10.,-1.10900986674273,0.7));
#11055=CARTESIAN_POINT('Ctrl Pts',(9.42188472144661,-1.13881853066854,0.7));
#11056=CARTESIAN_POINT('Ctrl Pts',(8.84359655223373,-1.16547286639245,0.7));
#11057=CARTESIAN_POINT('Ctrl Pts',(8.26514054272776,-1.18768929227839,0.7));
#11058=CARTESIAN_POINT('',(7.95,-1.,0.7));
#11059=CARTESIAN_POINT('Origin',(8.1,-1.,0.7));
#11060=CARTESIAN_POINT('',(7.95,1.,0.7));
#11061=CARTESIAN_POINT('Origin',(8.1,1.,0.7));
#11062=CARTESIAN_POINT('',(8.4,-4.89858719658942E-17,0.7));
#11063=CARTESIAN_POINT('Origin',(8.8,0.,0.7));
#11064=CARTESIAN_POINT('Origin',(8.97320508075689,0.3,0.9));
#11065=CARTESIAN_POINT('',(8.97320508075689,0.3,0.9));
#11066=CARTESIAN_POINT('',(9.14641016151377,0.,0.9));
#11067=CARTESIAN_POINT('',(8.59150635094611,0.961121593216771,0.9));
#11068=CARTESIAN_POINT('',(8.97320508075689,0.3,0.6));
#11069=CARTESIAN_POINT('',(8.97320508075689,0.3,0.9));
#11070=CARTESIAN_POINT('',(9.14641016151377,0.,0.6));
#11071=CARTESIAN_POINT('',(9.14641016151377,0.,0.6));
#11072=CARTESIAN_POINT('',(9.14641016151377,0.,0.9));
#11073=CARTESIAN_POINT('Origin',(8.62679491924311,0.3,0.9));
#11074=CARTESIAN_POINT('',(8.62679491924311,0.3,0.9));
#11075=CARTESIAN_POINT('',(7.01339745962156,0.3,0.9));
#11076=CARTESIAN_POINT('',(8.62679491924311,0.3,0.6));
#11077=CARTESIAN_POINT('',(8.62679491924311,0.3,0.9));
#11078=CARTESIAN_POINT('',(8.97320508075689,0.3,0.6));
#11079=CARTESIAN_POINT('Origin',(8.45358983848623,5.55111512312578E-17,
0.9));
#11080=CARTESIAN_POINT('',(8.45358983848623,4.24230095489963E-17,0.9));
#11081=CARTESIAN_POINT('',(8.07189110867545,-0.661121593216771,0.9));
#11082=CARTESIAN_POINT('',(8.45358983848623,5.55111512312578E-17,0.6));
#11083=CARTESIAN_POINT('',(8.45358983848623,4.24230095489963E-17,0.9));
#11084=CARTESIAN_POINT('',(8.62679491924311,0.3,0.6));
#11085=CARTESIAN_POINT('Origin',(8.62679491924311,-0.3,0.9));
#11086=CARTESIAN_POINT('',(8.62679491924311,-0.3,0.9));
#11087=CARTESIAN_POINT('',(8.15849364905389,0.511121593216771,0.9));
#11088=CARTESIAN_POINT('',(8.62679491924311,-0.3,0.6));
#11089=CARTESIAN_POINT('',(8.62679491924311,-0.3,0.9));
#11090=CARTESIAN_POINT('',(8.45358983848623,4.24230095489963E-17,0.6));
#11091=CARTESIAN_POINT('Origin',(8.97320508075689,-0.3,0.9));
#11092=CARTESIAN_POINT('',(8.97320508075689,-0.3,0.9));
#11093=CARTESIAN_POINT('',(7.18660254037844,-0.3,0.9));
#11094=CARTESIAN_POINT('',(8.97320508075689,-0.3,0.6));
#11095=CARTESIAN_POINT('',(8.97320508075689,-0.3,0.9));
#11096=CARTESIAN_POINT('',(8.62679491924311,-0.3,0.6));
#11097=CARTESIAN_POINT('Origin',(9.14641016151377,0.,0.9));
#11098=CARTESIAN_POINT('',(8.67810889132456,-0.811121593216771,0.9));
#11099=CARTESIAN_POINT('',(8.97320508075689,-0.3,0.6));
#11100=CARTESIAN_POINT('Origin',(8.8,5.55111512312578E-17,0.6));
#11101=CARTESIAN_POINT('',(8.63,-2.0818995585505E-17,0.6));
#11102=CARTESIAN_POINT('Origin',(8.8,0.,0.6));
#11103=CARTESIAN_POINT('Origin',(2.17320508075689,0.3,0.9));
#11104=CARTESIAN_POINT('',(2.17320508075689,0.3,0.9));
#11105=CARTESIAN_POINT('',(2.34641016151378,0.,0.9));
#11106=CARTESIAN_POINT('',(2.64150635094611,-0.511121593216773,0.9));
#11107=CARTESIAN_POINT('',(2.17320508075689,0.3,0.6));
#11108=CARTESIAN_POINT('',(2.17320508075689,0.3,0.9));
#11109=CARTESIAN_POINT('',(2.34641016151378,0.,0.6));
#11110=CARTESIAN_POINT('',(2.34641016151378,0.,0.6));
#11111=CARTESIAN_POINT('',(2.34641016151378,0.,0.9));
#11112=CARTESIAN_POINT('Origin',(1.82679491924311,0.3,0.9));
#11113=CARTESIAN_POINT('',(1.82679491924311,0.3,0.9));
#11114=CARTESIAN_POINT('',(3.61339745962156,0.3,0.9));
#11115=CARTESIAN_POINT('',(1.82679491924311,0.3,0.6));
#11116=CARTESIAN_POINT('',(1.82679491924311,0.3,0.9));
#11117=CARTESIAN_POINT('',(2.17320508075689,0.3,0.6));
#11118=CARTESIAN_POINT('Origin',(1.65358983848622,5.55111512312578E-17,
0.9));
#11119=CARTESIAN_POINT('',(1.65358983848622,4.24230095489963E-17,0.9));
#11120=CARTESIAN_POINT('',(2.12189110867545,0.811121593216773,0.9));
#11121=CARTESIAN_POINT('',(1.65358983848622,5.55111512312578E-17,0.6));
#11122=CARTESIAN_POINT('',(1.65358983848622,4.24230095489963E-17,0.9));
#11123=CARTESIAN_POINT('',(1.82679491924311,0.3,0.6));
#11124=CARTESIAN_POINT('Origin',(1.82679491924311,-0.3,0.9));
#11125=CARTESIAN_POINT('',(1.82679491924311,-0.3,0.9));
#11126=CARTESIAN_POINT('',(2.20849364905389,-0.961121593216772,0.9));
#11127=CARTESIAN_POINT('',(1.82679491924311,-0.3,0.6));
#11128=CARTESIAN_POINT('',(1.82679491924311,-0.3,0.9));
#11129=CARTESIAN_POINT('',(1.65358983848622,4.24230095489963E-17,0.6));
#11130=CARTESIAN_POINT('Origin',(2.17320508075689,-0.3,0.9));
#11131=CARTESIAN_POINT('',(2.17320508075689,-0.3,0.9));
#11132=CARTESIAN_POINT('',(3.78660254037844,-0.3,0.9));
#11133=CARTESIAN_POINT('',(2.17320508075689,-0.3,0.6));
#11134=CARTESIAN_POINT('',(2.17320508075689,-0.3,0.9));
#11135=CARTESIAN_POINT('',(1.82679491924311,-0.3,0.6));
#11136=CARTESIAN_POINT('Origin',(2.34641016151378,0.,0.9));
#11137=CARTESIAN_POINT('',(2.72810889132455,0.661121593216773,0.9));
#11138=CARTESIAN_POINT('',(2.17320508075689,-0.3,0.6));
#11139=CARTESIAN_POINT('Origin',(2.,5.55111512312578E-17,0.6));
#11140=CARTESIAN_POINT('',(1.83,-2.0818995585505E-17,0.6));
#11141=CARTESIAN_POINT('Origin',(2.,0.,0.6));
#11142=CARTESIAN_POINT('Origin',(8.1,-1.,0.8));
#11143=CARTESIAN_POINT('',(7.95,-1.,0.9));
#11144=CARTESIAN_POINT('Origin',(8.1,-1.,0.9));
#11145=CARTESIAN_POINT('',(7.95,-1.,0.8));
#11146=CARTESIAN_POINT('Origin',(2.7,-1.,0.8));
#11147=CARTESIAN_POINT('',(2.55,-1.,0.9));
#11148=CARTESIAN_POINT('Origin',(2.7,-1.,0.9));
#11149=CARTESIAN_POINT('',(2.55,-1.,0.7));
#11150=CARTESIAN_POINT('',(2.55,-1.,0.8));
#11151=CARTESIAN_POINT('Origin',(2.7,-1.,0.7));
#11152=CARTESIAN_POINT('Origin',(2.7,1.,0.8));
#11153=CARTESIAN_POINT('',(2.55,1.,0.9));
#11154=CARTESIAN_POINT('Origin',(2.7,1.,0.9));
#11155=CARTESIAN_POINT('',(2.55,1.,0.7));
#11156=CARTESIAN_POINT('',(2.55,1.,0.8));
#11157=CARTESIAN_POINT('Origin',(2.7,1.,0.7));
#11158=CARTESIAN_POINT('Origin',(8.1,1.,0.8));
#11159=CARTESIAN_POINT('',(7.95,1.,0.9));
#11160=CARTESIAN_POINT('Origin',(8.1,1.,0.9));
#11161=CARTESIAN_POINT('',(7.95,1.,0.8));
#11162=CARTESIAN_POINT('Origin',(2.,0.,0.45));
#11163=CARTESIAN_POINT('',(1.83,-2.0818995585505E-17,0.32));
#11164=CARTESIAN_POINT('',(1.83,2.0818995585505E-17,0.45));
#11165=CARTESIAN_POINT('Origin',(2.,0.,0.32));
#11166=CARTESIAN_POINT('Origin',(8.8,0.,0.45));
#11167=CARTESIAN_POINT('',(8.63,-2.0818995585505E-17,0.32));
#11168=CARTESIAN_POINT('',(8.63,2.0818995585505E-17,0.45));
#11169=CARTESIAN_POINT('Origin',(8.8,0.,0.32));
#11170=CARTESIAN_POINT('Origin',(10.,-0.62,0.32));
#11171=CARTESIAN_POINT('',(0.200274469199584,-0.62,0.));
#11172=CARTESIAN_POINT('',(0.217044958570157,-0.62,0.32));
#11173=CARTESIAN_POINT('',(0.221783445591644,-0.62,0.410415718550007));
#11174=CARTESIAN_POINT('',(0.,-0.62,0.));
#11175=CARTESIAN_POINT('',(7.7,-0.62,0.));
#11176=CARTESIAN_POINT('',(0.0167704893705732,-0.62,0.32));
#11177=CARTESIAN_POINT('',(0.0220575386407278,-0.62,0.420882909798596));
#11178=CARTESIAN_POINT('',(-0.1,-0.62,0.32));
#11179=CARTESIAN_POINT('Origin',(10.,-0.62,0.32));
#11180=CARTESIAN_POINT('',(0.9,-0.62,0.32));
#11181=CARTESIAN_POINT('',(0.9,-0.62,0.));
#11182=CARTESIAN_POINT('',(0.9,-0.62,0.16));
#11183=CARTESIAN_POINT('',(1.1,-0.62,0.32));
#11184=CARTESIAN_POINT('',(-0.1,-0.62,0.32));
#11185=CARTESIAN_POINT('',(1.1,-0.62,0.));
#11186=CARTESIAN_POINT('',(1.1,-0.62,0.16));
#11187=CARTESIAN_POINT('',(7.7,-0.62,0.));
#11188=CARTESIAN_POINT('Origin',(10.,-0.62,0.32));
#11189=CARTESIAN_POINT('',(3.5,-0.62,0.32));
#11190=CARTESIAN_POINT('',(3.5,-0.62,0.));
#11191=CARTESIAN_POINT('',(3.5,-0.62,0.16));
#11192=CARTESIAN_POINT('',(3.7,-0.62,0.32));
#11193=CARTESIAN_POINT('',(-0.1,-0.62,0.32));
#11194=CARTESIAN_POINT('',(3.7,-0.62,0.));
#11195=CARTESIAN_POINT('',(3.7,-0.62,0.16));
#11196=CARTESIAN_POINT('',(7.7,-0.62,0.));
#11197=CARTESIAN_POINT('Origin',(10.,-0.62,0.32));
#11198=CARTESIAN_POINT('',(7.1,-0.62,0.32));
#11199=CARTESIAN_POINT('',(7.1,-0.62,0.));
#11200=CARTESIAN_POINT('',(7.1,-0.62,0.16));
#11201=CARTESIAN_POINT('',(7.3,-0.62,0.32));
#11202=CARTESIAN_POINT('',(-0.1,-0.62,0.32));
#11203=CARTESIAN_POINT('',(7.3,-0.62,0.));
#11204=CARTESIAN_POINT('',(7.3,-0.62,0.16));
#11205=CARTESIAN_POINT('',(7.7,-0.62,0.));
#11206=CARTESIAN_POINT('Origin',(-0.0999999999999996,0.62,0.32));
#11207=CARTESIAN_POINT('',(0.217044958570158,0.62,0.32));
#11208=CARTESIAN_POINT('',(0.200274469199584,0.62,0.));
#11209=CARTESIAN_POINT('',(0.207951231396534,0.62,0.146481348799182));
#11210=CARTESIAN_POINT('',(0.0167704893705736,0.62,0.32));
#11211=CARTESIAN_POINT('',(10.,0.62,0.32));
#11212=CARTESIAN_POINT('',(0.,0.62,0.));
#11213=CARTESIAN_POINT('',(0.00822532444561912,0.62,0.156948540047771));
#11214=CARTESIAN_POINT('',(2.65,0.62,0.));
#11215=CARTESIAN_POINT('Origin',(-0.0999999999999996,0.62,0.32));
#11216=CARTESIAN_POINT('',(0.9,0.62,0.));
#11217=CARTESIAN_POINT('',(0.9,0.62,0.32));
#11218=CARTESIAN_POINT('',(0.9,0.62,0.16));
#11219=CARTESIAN_POINT('',(1.1,0.62,0.));
#11220=CARTESIAN_POINT('',(2.65,0.62,0.));
#11221=CARTESIAN_POINT('',(1.1,0.62,0.32));
#11222=CARTESIAN_POINT('',(1.1,0.62,0.16));
#11223=CARTESIAN_POINT('',(10.,0.62,0.32));
#11224=CARTESIAN_POINT('Origin',(-0.0999999999999996,0.62,0.32));
#11225=CARTESIAN_POINT('',(3.5,0.62,0.));
#11226=CARTESIAN_POINT('',(3.5,0.62,0.32));
#11227=CARTESIAN_POINT('',(3.5,0.62,0.16));
#11228=CARTESIAN_POINT('',(3.7,0.62,0.));
#11229=CARTESIAN_POINT('',(2.65,0.62,0.));
#11230=CARTESIAN_POINT('',(3.7,0.62,0.32));
#11231=CARTESIAN_POINT('',(3.7,0.62,0.16));
#11232=CARTESIAN_POINT('',(10.,0.62,0.32));
#11233=CARTESIAN_POINT('Origin',(4.95,0.,0.32));
#11234=CARTESIAN_POINT('',(1.6,-4.89858719658941E-17,0.32));
#11235=CARTESIAN_POINT('Origin',(2.,0.,0.32));
#11236=CARTESIAN_POINT('Origin',(4.95,0.,0.32));
#11237=CARTESIAN_POINT('',(8.4,-4.89858719658942E-17,0.32));
#11238=CARTESIAN_POINT('Origin',(8.8,0.,0.32));
#11239=CARTESIAN_POINT('Origin',(4.95,0.,0.32));
#11240=CARTESIAN_POINT('',(0.217044958570157,-0.7,0.32));
#11241=CARTESIAN_POINT('',(0.0167704893705731,-0.7,0.32));
#11242=CARTESIAN_POINT('Origin',(4.95,0.,0.32));
#11243=CARTESIAN_POINT('',(0.9,0.671641708581009,0.32));
#11244=CARTESIAN_POINT('',(1.1,-0.671641708581009,0.32));
#11245=CARTESIAN_POINT('Origin',(4.95,0.,0.32));
#11246=CARTESIAN_POINT('',(3.5,0.723888888888889,0.32));
#11247=CARTESIAN_POINT('',(3.7,-0.723888888888889,0.32));
#11248=CARTESIAN_POINT('Origin',(4.95,0.,0.32));
#11249=CARTESIAN_POINT('',(7.1,0.62,0.32));
#11250=CARTESIAN_POINT('',(7.1,0.712777777777778,0.32));
#11251=CARTESIAN_POINT('',(7.3,0.62,0.32));
#11252=CARTESIAN_POINT('',(10.,0.62,0.32));
#11253=CARTESIAN_POINT('',(7.3,-0.712777777777778,0.32));
#11254=CARTESIAN_POINT('Origin',(-0.0999999999999996,0.62,0.32));
#11255=CARTESIAN_POINT('',(7.1,0.62,0.));
#11256=CARTESIAN_POINT('',(7.1,0.62,0.16));
#11257=CARTESIAN_POINT('',(7.3,0.62,0.));
#11258=CARTESIAN_POINT('',(2.65,0.62,0.));
#11259=CARTESIAN_POINT('',(7.3,0.62,0.16));
#11260=CARTESIAN_POINT('Origin',(10.,1.30754691548544,0.));
#11261=CARTESIAN_POINT('',(10.,1.24211782565704,0.));
#11262=CARTESIAN_POINT('',(10.,-1.24211782565704,0.));
#11263=CARTESIAN_POINT('',(10.,1.30754691548544,0.));
#11264=CARTESIAN_POINT('',(10.,-1.20899340483173,0.605457329065657));
#11265=CARTESIAN_POINT('Ctrl Pts',(10.,-1.20899340483173,0.605457329065657));
#11266=CARTESIAN_POINT('Ctrl Pts',(10.,-1.21451837038612,0.504502771559899));
#11267=CARTESIAN_POINT('Ctrl Pts',(10.,-1.22004249263249,0.403547366186347));
#11268=CARTESIAN_POINT('Ctrl Pts',(10.,-1.23108392958594,0.201728789021226));
#11269=CARTESIAN_POINT('Ctrl Pts',(10.,-1.23660133320922,0.100864020914724));
#11270=CARTESIAN_POINT('Ctrl Pts',(10.,-1.24211782565704,0.));
#11271=CARTESIAN_POINT('Ctrl Pts',(10.,-1.10900986674273,0.7));
#11272=CARTESIAN_POINT('Ctrl Pts',(10.,-1.11692706738765,0.7));
#11273=CARTESIAN_POINT('Ctrl Pts',(9.99999896020971,-1.12478097169818,0.699006158364426));
#11274=CARTESIAN_POINT('Ctrl Pts',(9.99999805494427,-1.13243115645175,0.697118998397561));
#11275=CARTESIAN_POINT('Ctrl Pts',(9.99999754769332,-1.13671781459207,0.696061558623929));
#11276=CARTESIAN_POINT('Ctrl Pts',(9.99999708556116,-1.14094056283945,0.694722610426682));
#11277=CARTESIAN_POINT('Ctrl Pts',(9.99999679002998,-1.14507302265453,0.693112977943955));
#11278=CARTESIAN_POINT('Ctrl Pts',(9.99999625879002,-1.15250143622127,0.690219540062595));
#11279=CARTESIAN_POINT('Ctrl Pts',(9.999996365957,-1.15955821040664,0.686485807665162));
#11280=CARTESIAN_POINT('Ctrl Pts',(9.99999703387985,-1.16609707610076,0.681992895329386));
#11281=CARTESIAN_POINT('Ctrl Pts',(9.99999740034986,-1.16968476316425,0.679527763880215));
#11282=CARTESIAN_POINT('Ctrl Pts',(9.99999792190556,-1.17311627083768,0.676833210412541));
#11283=CARTESIAN_POINT('Ctrl Pts',(9.99999838578331,-1.17636354905877,0.673917165661822));
#11284=CARTESIAN_POINT('Ctrl Pts',(9.99999884023993,-1.17954487655573,0.671060344436104));
#11285=CARTESIAN_POINT('Ctrl Pts',(9.99999924462882,-1.18253006594632,0.668008218820746));
#11286=CARTESIAN_POINT('Ctrl Pts',(9.99999924442301,-1.185296421281,0.664772262763763));
#11287=CARTESIAN_POINT('Ctrl Pts',(9.99999924404215,-1.19041578560695,0.658783864313737));
#11288=CARTESIAN_POINT('Ctrl Pts',(9.99999800949836,-1.19478865237554,0.652167294255586));
#11289=CARTESIAN_POINT('Ctrl Pts',(9.99999759228052,-1.19835462180986,0.645087621913151));
#11290=CARTESIAN_POINT('Ctrl Pts',(9.99999755030119,-1.19871341999785,0.644375284453517));
#11291=CARTESIAN_POINT('Ctrl Pts',(9.9999975145836,-1.19906401030029,0.643658239626438));
#11292=CARTESIAN_POINT('Ctrl Pts',(9.99999748581823,-1.19940630408966,0.642936645100882));
#11293=CARTESIAN_POINT('Ctrl Pts',(9.99999720003888,-1.20280693749908,0.635767720253638));
#11294=CARTESIAN_POINT('Ctrl Pts',(9.9999978299417,-1.20535324884233,0.628234501710241));
#11295=CARTESIAN_POINT('Ctrl Pts',(9.99999874867777,-1.20699142055415,0.62050509267719));
#11296=CARTESIAN_POINT('Ctrl Pts',(9.99999933690345,-1.20804026874419,0.615556297251186));
#11297=CARTESIAN_POINT('Ctrl Pts',(9.99999999916487,-1.20871598809812,0.61052641213707));
#11298=CARTESIAN_POINT('Ctrl Pts',(9.99999999968202,-1.20899340489109,0.605457329065633));
#11299=CARTESIAN_POINT('Ctrl Pts',(10.,1.24211782565704,0.));
#11300=CARTESIAN_POINT('Ctrl Pts',(10.,1.23660053043673,0.100878698875723));
#11301=CARTESIAN_POINT('Ctrl Pts',(10.,1.23108232376984,0.201758145268796));
#11302=CARTESIAN_POINT('Ctrl Pts',(10.,1.22004088630648,0.403576722396156));
#11303=CARTESIAN_POINT('Ctrl Pts',(10.,1.2145175671044,0.504517449470448));
#11304=CARTESIAN_POINT('Ctrl Pts',(10.,1.20899340483173,0.605457329065657));
#11305=CARTESIAN_POINT('Origin',(7.3,-1.42555555555556,0.));
#11306=CARTESIAN_POINT('',(7.3,1.35236351479115,0.));
#11307=CARTESIAN_POINT('',(7.3,-1.42555555555556,0.));
#11308=CARTESIAN_POINT('Ctrl Pts',(7.29999999953133,1.3203161347307,0.605285370449834));
#11309=CARTESIAN_POINT('Ctrl Pts',(7.29999999953133,1.32565322760551,0.504490726585133));
#11310=CARTESIAN_POINT('Ctrl Pts',(7.3,1.33099015509697,0.403695123734478));
#11311=CARTESIAN_POINT('Ctrl Pts',(7.3,1.34167258064689,0.201933969199042));
#11312=CARTESIAN_POINT('Ctrl Pts',(7.3,1.34701817868136,0.100966514951419));
#11313=CARTESIAN_POINT('Ctrl Pts',(7.3,1.35236351479115,0.));
#11314=CARTESIAN_POINT('',(7.29999999953133,-1.3203161347307,0.605285370449834));
#11315=CARTESIAN_POINT('Ctrl Pts',(7.3,-1.32031613470337,0.605285370449877));
#11316=CARTESIAN_POINT('Ctrl Pts',(7.3,-1.31989712778929,0.61319860217968));
#11317=CARTESIAN_POINT('Ctrl Pts',(7.29999916171872,-1.31851071739963,0.621020829077898));
#11318=CARTESIAN_POINT('Ctrl Pts',(7.29999878808195,-1.31624092632926,0.628591660945423));
#11319=CARTESIAN_POINT('Ctrl Pts',(7.29999857947278,-1.31497365483497,0.632818613610392));
#11320=CARTESIAN_POINT('Ctrl Pts',(7.29999848639856,-1.31343001415,0.636967235874856));
#11321=CARTESIAN_POINT('Ctrl Pts',(7.29999853830689,-1.31161789606625,0.641007613679984));
#11322=CARTESIAN_POINT('Ctrl Pts',(7.29999863125487,-1.30837308502546,0.648242386418365));
#11323=CARTESIAN_POINT('Ctrl Pts',(7.29999925734287,-1.30430566789097,0.655052076019481));
#11324=CARTESIAN_POINT('Ctrl Pts',(7.29999949821933,-1.29947941328181,0.661273460789274));
#11325=CARTESIAN_POINT('Ctrl Pts',(7.29999954322,-1.29857776968225,0.662435743389828));
#11326=CARTESIAN_POINT('Ctrl Pts',(7.29999957102613,-1.29764951297213,0.663577423078133));
#11327=CARTESIAN_POINT('Ctrl Pts',(7.2999995707084,-1.29669488998092,0.664697318929248));
#11328=CARTESIAN_POINT('Ctrl Pts',(7.29999957007561,-1.29479368240016,0.666927680549918));
#11329=CARTESIAN_POINT('Ctrl Pts',(7.29999945886743,-1.29278792931167,0.669071688571899));
#11330=CARTESIAN_POINT('Ctrl Pts',(7.29999930790078,-1.2906849717248,0.671125563583336));
#11331=CARTESIAN_POINT('Ctrl Pts',(7.29999889984047,-1.28500071247856,0.676677153447665));
#11332=CARTESIAN_POINT('Ctrl Pts',(7.29999826931494,-1.27867319504519,0.681510485910933));
#11333=CARTESIAN_POINT('Ctrl Pts',(7.29999806345125,-1.27186607945067,0.685571085769401));
#11334=CARTESIAN_POINT('Ctrl Pts',(7.29999793266427,-1.26754145993833,0.688150820039508));
#11335=CARTESIAN_POINT('Ctrl Pts',(7.29999794545359,-1.26302231037287,0.690417984675215));
#11336=CARTESIAN_POINT('Ctrl Pts',(7.29999810371711,-1.25834494218995,0.69234933099425));
#11337=CARTESIAN_POINT('Ctrl Pts',(7.29999835129001,-1.25102809722258,0.695370551698293));
#11338=CARTESIAN_POINT('Ctrl Pts',(7.29999895574222,-1.24340909242398,0.6975375590939));
#11339=CARTESIAN_POINT('Ctrl Pts',(7.29999944081525,-1.2356348173965,0.698780605629559));
#11340=CARTESIAN_POINT('Ctrl Pts',(7.29999975409932,-1.23061380764338,0.699583426311495));
#11341=CARTESIAN_POINT('Ctrl Pts',(7.30000000047446,-1.22552743956586,0.699999999832051));
#11342=CARTESIAN_POINT('Ctrl Pts',(7.29999999989087,-1.22041345054982,0.7));
#11343=CARTESIAN_POINT('',(7.3,-1.35236351479115,0.));
#11344=CARTESIAN_POINT('Ctrl Pts',(7.3,-1.35236351479115,0.));
#11345=CARTESIAN_POINT('Ctrl Pts',(7.3,-1.34701814920095,0.100967071798286));
#11346=CARTESIAN_POINT('Ctrl Pts',(7.3,-1.34167252169398,0.201935082699409));
#11347=CARTESIAN_POINT('Ctrl Pts',(7.3,-1.33099009614589,0.403696237111114));
#11348=CARTESIAN_POINT('Ctrl Pts',(7.29999999953133,-1.32565319812959,0.504491283257837));
#11349=CARTESIAN_POINT('Ctrl Pts',(7.29999999953133,-1.3203161347307,0.605285370449834));
#11350=CARTESIAN_POINT('',(7.3,-1.42555555555556,0.));
#11351=CARTESIAN_POINT('Origin',(3.7,-1.44777777777778,0.));
#11352=CARTESIAN_POINT('',(3.7,1.37924639543935,0.));
#11353=CARTESIAN_POINT('',(3.7,-1.44777777777778,0.));
#11354=CARTESIAN_POINT('',(3.7,1.34735368793805,0.605261457205193));
#11355=CARTESIAN_POINT('Ctrl Pts',(3.7,1.34735368793805,0.605261457205193));
#11356=CARTESIAN_POINT('Ctrl Pts',(3.7,1.35266395147774,0.504488703431434));
#11357=CARTESIAN_POINT('Ctrl Pts',(3.7,1.35797406404029,0.40371594170176));
#11358=CARTESIAN_POINT('Ctrl Pts',(3.7,1.36860496587027,0.201962122597264));
#11359=CARTESIAN_POINT('Ctrl Pts',(3.7,1.37392575452088,0.100981065191366));
#11360=CARTESIAN_POINT('Ctrl Pts',(3.7,1.37924639543935,0.));
#11361=CARTESIAN_POINT('',(3.7,1.24747724070879,0.7));
#11362=CARTESIAN_POINT('Ctrl Pts',(3.7,1.24747724070879,0.7));
#11363=CARTESIAN_POINT('Ctrl Pts',(3.7,1.25538532734776,0.7));
#11364=CARTESIAN_POINT('Ctrl Pts',(3.70000034866643,1.26322972530331,0.699006048248363));
#11365=CARTESIAN_POINT('Ctrl Pts',(3.70000065268588,1.27087026624727,0.697119044026295));
#11366=CARTESIAN_POINT('Ctrl Pts',(3.7000008238479,1.27517186762995,0.696056666371322));
#11367=CARTESIAN_POINT('Ctrl Pts',(3.70000097972585,1.27940891103121,0.694710185093394));
#11368=CARTESIAN_POINT('Ctrl Pts',(3.70000107833511,1.28355469746902,0.693090631030141));
#11369=CARTESIAN_POINT('Ctrl Pts',(3.70000125487464,1.29097687270382,0.690191153635441));
#11370=CARTESIAN_POINT('Ctrl Pts',(3.7000012145424,1.29802606517866,0.686451118058958));
#11371=CARTESIAN_POINT('Ctrl Pts',(3.70000098691147,1.3045562506385,0.681952404110064));
#11372=CARTESIAN_POINT('Ctrl Pts',(3.70000086156653,1.30815209635338,0.679475187900035));
#11373=CARTESIAN_POINT('Ctrl Pts',(3.70000068390876,1.31159030769532,0.676767042898431));
#11374=CARTESIAN_POINT('Ctrl Pts',(3.70000052608992,1.31484259178137,0.673836088143417));
#11375=CARTESIAN_POINT('Ctrl Pts',(3.70000037216713,1.31801458722906,0.670977489418868));
#11376=CARTESIAN_POINT('Ctrl Pts',(3.70000023558528,1.32099045552882,0.667924239810466));
#11377=CARTESIAN_POINT('Ctrl Pts',(3.70000023595245,1.32374763345498,0.664687876924229));
#11378=CARTESIAN_POINT('Ctrl Pts',(3.70000023663259,1.32885491153898,0.658692977181302));
#11379=CARTESIAN_POINT('Ctrl Pts',(3.70000065621025,1.33321474659758,0.652071180203097));
#11380=CARTESIAN_POINT('Ctrl Pts',(3.70000080093706,1.33676785491319,0.644988218508662));
#11381=CARTESIAN_POINT('Ctrl Pts',(3.70000081573428,1.33713113341147,0.644264039153811));
#11382=CARTESIAN_POINT('Ctrl Pts',(3.70000082835625,1.33748593861467,0.643535019157411));
#11383=CARTESIAN_POINT('Ctrl Pts',(3.70000083855542,1.33783217873901,0.642801324492746));
#11384=CARTESIAN_POINT('Ctrl Pts',(3.70000093832019,1.34121897990539,0.63562457699476));
#11385=CARTESIAN_POINT('Ctrl Pts',(3.70000072997693,1.34375116782692,0.628085030530103));
#11386=CARTESIAN_POINT('Ctrl Pts',(3.70000042189378,1.34537558692779,0.6203512574804));
#11387=CARTESIAN_POINT('Ctrl Pts',(3.70000022417294,1.3464181026242,0.615387895628485));
#11388=CARTESIAN_POINT('Ctrl Pts',(3.70000000036652,1.34708586836718,0.6103438638189));
#11389=CARTESIAN_POINT('Ctrl Pts',(3.69999999992214,1.34735368792773,0.6052614572053));
#11390=CARTESIAN_POINT('',(3.7,-1.24747724070944,0.7));
#11391=CARTESIAN_POINT('',(3.7,-0.723888888888889,0.7));
#11392=CARTESIAN_POINT('',(3.7,-1.34735368793805,0.605261457205193));
#11393=CARTESIAN_POINT('Ctrl Pts',(3.69999999992215,-1.34735368792773,0.6052614572053));
#11394=CARTESIAN_POINT('Ctrl Pts',(3.70000000061408,-1.34693666923469,0.613175212866596));
#11395=CARTESIAN_POINT('Ctrl Pts',(3.70000049671034,-1.34555248374866,0.620998392122869));
#11396=CARTESIAN_POINT('Ctrl Pts',(3.70000071566022,-1.34328499565267,0.628570462735333));
#11397=CARTESIAN_POINT('Ctrl Pts',(3.70000083807517,-1.34201724238155,0.632804009674372));
#11398=CARTESIAN_POINT('Ctrl Pts',(3.7000008913247,-1.34047237297042,0.63695909738719));
#11399=CARTESIAN_POINT('Ctrl Pts',(3.70000085837557,-1.33865827982058,0.641005656934072));
#11400=CARTESIAN_POINT('Ctrl Pts',(3.7000007994669,-1.33541492172585,0.648240369034365));
#11401=CARTESIAN_POINT('Ctrl Pts',(3.70000042420685,-1.33134915897915,0.655050234746405));
#11402=CARTESIAN_POINT('Ctrl Pts',(3.70000027984635,-1.32652447879733,0.661271863919233));
#11403=CARTESIAN_POINT('Ctrl Pts',(3.70000025294096,-1.32562527203035,0.662431429080655));
#11404=CARTESIAN_POINT('Ctrl Pts',(3.7000002362737,-1.32469957579387,0.663570491348455));
#11405=CARTESIAN_POINT('Ctrl Pts',(3.70000023630138,-1.32374763346102,0.664687876924223));
#11406=CARTESIAN_POINT('Ctrl Pts',(3.70000023635686,-1.32184039796576,0.666926581264246));
#11407=CARTESIAN_POINT('Ctrl Pts',(3.70000030283857,-1.31982784222224,0.669078323867587));
#11408=CARTESIAN_POINT('Ctrl Pts',(3.70000039320883,-1.31771738411303,0.671139279696989));
#11409=CARTESIAN_POINT('Ctrl Pts',(3.70000063660146,-1.3120333248939,0.676690015307994));
#11410=CARTESIAN_POINT('Ctrl Pts',(3.7000010126336,-1.30570602994251,0.681522474044465));
#11411=CARTESIAN_POINT('Ctrl Pts',(3.70000113724274,-1.29889910811053,0.685582059356066));
#11412=CARTESIAN_POINT('Ctrl Pts',(3.70000121634872,-1.29457784995583,0.688159217808216));
#11413=CARTESIAN_POINT('Ctrl Pts',(3.70000121058612,-1.2900623422215,0.690424215862126));
#11414=CARTESIAN_POINT('Ctrl Pts',(3.70000111831253,-1.28538881676413,0.692353818784707));
#11415=CARTESIAN_POINT('Ctrl Pts',(3.70000097388434,-1.27807373536961,0.695374066040565));
#11416=CARTESIAN_POINT('Ctrl Pts',(3.70000061691996,-1.27045659963863,0.697540160564298));
#11417=CARTESIAN_POINT('Ctrl Pts',(3.7000003304055,-1.26268427129293,0.698782316368755));
#11418=CARTESIAN_POINT('Ctrl Pts',(3.70000014548661,-1.25766794365683,0.699584014420239));
#11419=CARTESIAN_POINT('Ctrl Pts',(3.7,-1.25258637988459,0.7));
#11420=CARTESIAN_POINT('Ctrl Pts',(3.7,-1.24747724070879,0.7));
#11421=CARTESIAN_POINT('',(3.7,-1.37924639543935,0.));
#11422=CARTESIAN_POINT('Ctrl Pts',(3.7,-1.37924639543935,0.));
#11423=CARTESIAN_POINT('Ctrl Pts',(3.7,-1.37392574223662,0.100981298335747));
#11424=CARTESIAN_POINT('Ctrl Pts',(3.7,-1.36860494130098,0.201962588887634));
#11425=CARTESIAN_POINT('Ctrl Pts',(3.7,-1.35797403946962,0.403716407992068));
#11426=CARTESIAN_POINT('Ctrl Pts',(3.7,-1.3526639391921,0.504488936575732));
#11427=CARTESIAN_POINT('Ctrl Pts',(3.7,-1.34735368793805,0.605261457205193));
#11428=CARTESIAN_POINT('',(3.7,-1.44777777777778,0.));
#11429=CARTESIAN_POINT('Origin',(1.1,-1.34328341716202,0.));
#11430=CARTESIAN_POINT('',(1.1,1.27885335043294,0.));
#11431=CARTESIAN_POINT('',(1.1,-1.34328341716202,0.));
#11432=CARTESIAN_POINT('Ctrl Pts',(1.1,1.24553911298206,0.605485603995113));
#11433=CARTESIAN_POINT('Ctrl Pts',(1.1,1.25109559382646,0.504544105903265));
#11434=CARTESIAN_POINT('Ctrl Pts',(1.1,1.25665083308595,0.403601248768354));
#11435=CARTESIAN_POINT('Ctrl Pts',(1.1,1.26775551906787,0.201773573764085));
#11436=CARTESIAN_POINT('Ctrl Pts',(1.1,1.2733051088238,0.100886182270816));
#11437=CARTESIAN_POINT('Ctrl Pts',(1.1,1.27885335043294,0.));
#11438=CARTESIAN_POINT('',(1.1,-1.14549341399195,0.7));
#11439=CARTESIAN_POINT('',(1.1,-0.671641708581009,0.7));
#11440=CARTESIAN_POINT('',(1.1,-1.24553911298206,0.605485603995113));
#11441=CARTESIAN_POINT('Ctrl Pts',(1.09999999916631,-1.24553911263843,0.605485603997431));
#11442=CARTESIAN_POINT('Ctrl Pts',(1.10000000220634,-1.24510362317222,0.61339691285734));
#11443=CARTESIAN_POINT('Ctrl Pts',(1.10000177015643,-1.24370036622144,0.621215229994996));
#11444=CARTESIAN_POINT('Ctrl Pts',(1.10000252895322,-1.24141353486351,0.628780213666851));
#11445=CARTESIAN_POINT('Ctrl Pts',(1.10000294802756,-1.24015054543059,0.632958263090869));
#11446=CARTESIAN_POINT('Ctrl Pts',(1.10000312162076,-1.23861706177488,0.637059070655947));
#11447=CARTESIAN_POINT('Ctrl Pts',(1.10000299297862,-1.23682078380192,0.641053713130525));
#11448=CARTESIAN_POINT('Ctrl Pts',(1.10000275999609,-1.23356756237267,0.64828837095969));
#11449=CARTESIAN_POINT('Ctrl Pts',(1.10000138715103,-1.22949085733774,0.655096441442141));
#11450=CARTESIAN_POINT('Ctrl Pts',(1.10000084482056,-1.2246552743941,0.661315040399663));
#11451=CARTESIAN_POINT('Ctrl Pts',(1.10000074196669,-1.22373819809959,0.662494407966206));
#11452=CARTESIAN_POINT('Ctrl Pts',(1.1000006773267,-1.22279369438101,0.663652502541609));
#11453=CARTESIAN_POINT('Ctrl Pts',(1.10000067553493,-1.22182202641035,0.66478809188211));
#11454=CARTESIAN_POINT('Ctrl Pts',(1.10000067210542,-1.219962222636,0.666961646435043));
#11455=CARTESIAN_POINT('Ctrl Pts',(1.10000089707048,-1.21800293160495,0.669052796220007));
#11456=CARTESIAN_POINT('Ctrl Pts',(1.10000120920309,-1.21595100691259,0.671058078730413));
#11457=CARTESIAN_POINT('Ctrl Pts',(1.10000207391986,-1.21026645613745,0.676613414309409));
#11458=CARTESIAN_POINT('Ctrl Pts',(1.1000034579227,-1.20393786500476,0.681450029097565));
#11459=CARTESIAN_POINT('Ctrl Pts',(1.10000394126019,-1.19712964857754,0.685514663758263));
#11460=CARTESIAN_POINT('Ctrl Pts',(1.10000424974863,-1.19278432848208,0.688108902478585));
#11461=CARTESIAN_POINT('Ctrl Pts',(1.10000425197701,-1.18824265871575,0.690387991283085));
#11462=CARTESIAN_POINT('Ctrl Pts',(1.10000394032285,-1.18354156621637,0.692328715646671));
#11463=CARTESIAN_POINT('Ctrl Pts',(1.10000345443802,-1.17621232165581,0.695354404566264));
#11464=CARTESIAN_POINT('Ctrl Pts',(1.10000219938511,-1.16858027633095,0.697525330589554));
#11465=CARTESIAN_POINT('Ctrl Pts',(1.10000118192936,-1.16079305972554,0.698772417158578));
#11466=CARTESIAN_POINT('Ctrl Pts',(1.10000052251962,-1.15574619011492,0.699580649884844));
#11467=CARTESIAN_POINT('Ctrl Pts',(1.1,-1.15063354328712,0.7));
#11468=CARTESIAN_POINT('Ctrl Pts',(1.1,-1.14549341399196,0.7));
#11469=CARTESIAN_POINT('',(1.1,-1.27885335043294,0.));
#11470=CARTESIAN_POINT('Ctrl Pts',(1.1,-1.27885335043294,0.));
#11471=CARTESIAN_POINT('Ctrl Pts',(1.1,-1.27330503870861,0.100887457206881));
#11472=CARTESIAN_POINT('Ctrl Pts',(1.1,-1.26775537880223,0.201776123688554));
#11473=CARTESIAN_POINT('Ctrl Pts',(1.1,-1.25665069275548,0.403603798678134));
#11474=CARTESIAN_POINT('Ctrl Pts',(1.1,-1.25109552364596,0.504545380833391));
#11475=CARTESIAN_POINT('Ctrl Pts',(1.1,-1.24553911298206,0.605485603995113));
#11476=CARTESIAN_POINT('',(1.1,-1.34328341716202,0.));
#11477=CARTESIAN_POINT('Origin',(0.199725906950915,-1.4,-0.0104671912485888));
#11478=CARTESIAN_POINT('',(0.200274469199584,1.12301388185427,1.38777878078145E-17));
#11479=CARTESIAN_POINT('',(0.200274469199585,-0.7,0.));
#11480=CARTESIAN_POINT('',(0.231993417893744,1.09142177001972,0.605233595624295));
#11481=CARTESIAN_POINT('Ctrl Pts',(0.200274469199584,1.12301388185427,-2.97071395261028E-17));
#11482=CARTESIAN_POINT('Ctrl Pts',(0.210847451470635,1.11248294808,0.201744519910852));
#11483=CARTESIAN_POINT('Ctrl Pts',(0.22142043436526,1.101952242875,0.403489051720196));
#11484=CARTESIAN_POINT('Ctrl Pts',(0.231993417893744,1.09142177001972,0.605233595624295));
#11485=CARTESIAN_POINT('',(0.231993417893744,-1.09142177001972,0.605233595624295));
#11486=CARTESIAN_POINT('',(0.231993417893744,-0.7,0.605233595624295));
#11487=CARTESIAN_POINT('',(0.200274469199584,-1.12301388185427,-1.38777878078145E-17));
#11488=CARTESIAN_POINT('Ctrl Pts',(0.231993417893744,-1.09142177001972,
0.605233595624295));
#11489=CARTESIAN_POINT('Ctrl Pts',(0.22142043436526,-1.101952242875,0.403489051720196));
#11490=CARTESIAN_POINT('Ctrl Pts',(0.210847451470635,-1.11248294808,0.201744519910852));
#11491=CARTESIAN_POINT('Ctrl Pts',(0.200274469199584,-1.12301388185427,
-4.90059381963448E-17));
#11492=CARTESIAN_POINT('',(0.200274469199585,-0.7,0.));
#11493=CARTESIAN_POINT('Origin',(5.4,-1.11022302462516E-16,0.));
#11494=CARTESIAN_POINT('Ctrl Pts',(7.29999999999999,-1.35236351479115,1.04083408558608E-17));
#11495=CARTESIAN_POINT('Ctrl Pts',(8.20044803681595,-1.32637404707459,3.18306896032855E-8));
#11496=CARTESIAN_POINT('Ctrl Pts',(9.10060048441536,-1.28803709316692,1.03188250195688E-8));
#11497=CARTESIAN_POINT('Ctrl Pts',(10.0000000000405,-1.24211782537639,-8.23328475353175E-12));
#11498=CARTESIAN_POINT('Ctrl Pts',(10.0000000000405,1.24211782537639,-8.23320567538283E-12));
#11499=CARTESIAN_POINT('Ctrl Pts',(9.1006004808701,1.28803709334794,1.03184817085883E-8));
#11500=CARTESIAN_POINT('Ctrl Pts',(8.20044803144508,1.32637404722969,3.18291413954212E-8));
#11501=CARTESIAN_POINT('Ctrl Pts',(7.3,1.35236351479115,4.75121773919879E-17));
#11502=CARTESIAN_POINT('',(7.1,1.35793097395724,0.));
#11503=CARTESIAN_POINT('',(7.1,1.42555555555556,0.));
#11504=CARTESIAN_POINT('Ctrl Pts',(7.1000000000396,1.35793097389613,-4.88924676637329E-12));
#11505=CARTESIAN_POINT('Ctrl Pts',(6.53177385320612,1.37316067096195,3.71763852401782E-9));
#11506=CARTESIAN_POINT('Ctrl Pts',(5.96344379069665,1.38333257666104,-3.82408184804385E-8));
#11507=CARTESIAN_POINT('Ctrl Pts',(5.39512359652123,1.38725406840392,-3.97623797275691E-8));
#11508=CARTESIAN_POINT('Ctrl Pts',(4.82973248928002,1.39115534902226,-4.12760989429076E-8));
#11509=CARTESIAN_POINT('Ctrl Pts',(4.26470859812609,1.38886839226708,1.63957607983357E-8));
#11510=CARTESIAN_POINT('Ctrl Pts',(3.70000000036239,1.37924639538501,-6.25376529969227E-12));
#11511=CARTESIAN_POINT('',(3.5,1.37552980833516,0.));
#11512=CARTESIAN_POINT('',(3.5,1.44777777777778,0.));
#11513=CARTESIAN_POINT('Ctrl Pts',(3.50000000097466,1.37552980835479,1.06251812903579E-15));
#11514=CARTESIAN_POINT('Ctrl Pts',(2.69943075695685,1.35940904975719,2.35366119539541E-7));
#11515=CARTESIAN_POINT('Ctrl Pts',(1.89948254587541,1.32827224396921,2.51300192353997E-7));
#11516=CARTESIAN_POINT('Ctrl Pts',(1.10000000028363,1.27885335028943,-5.13283415455519E-11));
#11517=CARTESIAN_POINT('',(0.9,1.266106713614,0.));
#11518=CARTESIAN_POINT('',(0.9,1.34328341716202,0.));
#11519=CARTESIAN_POINT('',(0.292382661757373,1.22257596919059,0.));
#11520=CARTESIAN_POINT('Ctrl Pts',(0.9,1.266106713614,1.20346441145891E-16));
#11521=CARTESIAN_POINT('Ctrl Pts',(0.697432754539207,1.25280566772398,-2.10387859372414E-8));
#11522=CARTESIAN_POINT('Ctrl Pts',(0.494894520889663,1.23831317328004,3.6654767345328E-12));
#11523=CARTESIAN_POINT('Ctrl Pts',(0.292382661757371,1.22257596919059,2.98331735103528E-16));
#11524=CARTESIAN_POINT('Ctrl Pts',(0.292382661757373,1.22257596919059,2.94902990916057E-17));
#11525=CARTESIAN_POINT('Ctrl Pts',(0.284469747869226,1.22196105627757,-8.65621238729993E-13));
#11526=CARTESIAN_POINT('Ctrl Pts',(0.276673396002317,1.22038240716686,-1.19564355630166E-6));
#11527=CARTESIAN_POINT('Ctrl Pts',(0.269153172408756,1.21792571627104,-1.29137975931779E-6));
#11528=CARTESIAN_POINT('Ctrl Pts',(0.264330998492885,1.21635041859408,-1.35276844214688E-6));
#11529=CARTESIAN_POINT('Ctrl Pts',(0.259622238853914,1.21441292414196,-1.0165784587106E-6));
#11530=CARTESIAN_POINT('Ctrl Pts',(0.255072584042237,1.21212521597766,-4.21167369976509E-7));
#11531=CARTESIAN_POINT('Ctrl Pts',(0.247984787860257,1.20856125126747,5.06409032217246E-7));
#11532=CARTESIAN_POINT('Ctrl Pts',(0.241364979299678,1.20419126978451,2.25366520907849E-6));
#11533=CARTESIAN_POINT('Ctrl Pts',(0.235375785094684,1.19908071490398,1.28723124315333E-6));
#11534=CARTESIAN_POINT('Ctrl Pts',(0.235058634311792,1.19881009144014,1.23605486142058E-6));
#11535=CARTESIAN_POINT('Ctrl Pts',(0.234743258170683,1.19853738091759,1.17639378419006E-6));
#11536=CARTESIAN_POINT('Ctrl Pts',(0.234429683218046,1.19826258967301,1.10742116603597E-6));
#11537=CARTESIAN_POINT('Ctrl Pts',(0.23095881299434,1.19522100506769,3.4398325561458E-7));
#11538=CARTESIAN_POINT('Ctrl Pts',(0.227708211416394,1.19192479473749,-1.52348441667556E-6));
#11539=CARTESIAN_POINT('Ctrl Pts',(0.224692430858345,1.18840300965977,-3.42436181452249E-6));
#11540=CARTESIAN_POINT('Ctrl Pts',(0.219522873151367,1.18236607466387,-6.68278702580898E-6));
#11541=CARTESIAN_POINT('Ctrl Pts',(0.21509942609515,1.17573654654733,-9.78259773483875E-6));
#11542=CARTESIAN_POINT('Ctrl Pts',(0.211478909386775,1.16867548752938,-1.04320859863301E-5));
#11543=CARTESIAN_POINT('Ctrl Pts',(0.20968494559888,1.16517673715679,-1.075390701291E-5));
#11544=CARTESIAN_POINT('Ctrl Pts',(0.208088728862602,1.16157146972622,-1.05358292927083E-5));
#11545=CARTESIAN_POINT('Ctrl Pts',(0.206701335101202,1.15787708229469,-9.83193564179307E-6));
#11546=CARTESIAN_POINT('Ctrl Pts',(0.203919119965097,1.15046852899383,-8.42037994342582E-6));
#11547=CARTESIAN_POINT('Ctrl Pts',(0.202003457218558,1.1427818296106,-4.88542801801716E-6));
#11548=CARTESIAN_POINT('Ctrl Pts',(0.201024541128784,1.13496408391561,-2.30807221316776E-6));
#11549=CARTESIAN_POINT('Ctrl Pts',(0.200529226009753,1.13100843574523,-1.00397341389412E-6));
#11550=CARTESIAN_POINT('Ctrl Pts',(0.200274469344113,1.12701892049093,-1.14168925800036E-11));
#11551=CARTESIAN_POINT('Ctrl Pts',(0.200274469199584,1.12301388185427,-1.43114686768087E-17));
#11552=CARTESIAN_POINT('',(-1.73234772679968E-18,1.12356026268968,4.53319947845445E-20));
#11553=CARTESIAN_POINT('',(0.,-1.4,0.));
#11554=CARTESIAN_POINT('',(0.276326924564679,1.42224670711126,-2.77555756156289E-17));
#11555=CARTESIAN_POINT('Ctrl Pts',(0.276326924564681,1.42224670711126,-1.50920942409982E-16));
#11556=CARTESIAN_POINT('Ctrl Pts',(0.258529852003869,1.4208638358667,-3.32972379743633E-13));
#11557=CARTESIAN_POINT('Ctrl Pts',(0.240927013527826,1.41785398988725,-1.99727536601662E-6));
#11558=CARTESIAN_POINT('Ctrl Pts',(0.223720619657732,1.41333325652174,-2.71091968639774E-6));
#11559=CARTESIAN_POINT('Ctrl Pts',(0.206313289378911,1.40875972999491,-3.432897951005E-6));
#11560=CARTESIAN_POINT('Ctrl Pts',(0.18931019325249,1.40263932318529,-2.78724979559428E-6));
#11561=CARTESIAN_POINT('Ctrl Pts',(0.172932985028856,1.39504220432096,-6.31841720307455E-7));
#11562=CARTESIAN_POINT('Ctrl Pts',(0.170060146426803,1.39370954151055,-2.53746782677961E-7));
#11563=CARTESIAN_POINT('Ctrl Pts',(0.167206630967902,1.39233132643846,1.61597591574489E-7));
#11564=CARTESIAN_POINT('Ctrl Pts',(0.164373729059928,1.39090779908693,6.02790108062464E-7));
#11565=CARTESIAN_POINT('Ctrl Pts',(0.148213121449433,1.38278712717586,3.11962244863226E-6));
#11566=CARTESIAN_POINT('Ctrl Pts',(0.132864864406694,1.37326763401578,6.8005293729143E-6));
#11567=CARTESIAN_POINT('Ctrl Pts',(0.118540368157823,1.36244192017091,7.47011412280372E-6));
#11568=CARTESIAN_POINT('Ctrl Pts',(0.1130124780146,1.35826422653222,7.72851001154276E-6));
#11569=CARTESIAN_POINT('Ctrl Pts',(0.107637267132642,1.35389150739715,7.50091387420595E-6));
#11570=CARTESIAN_POINT('Ctrl Pts',(0.102427993107927,1.34932731552598,6.39696583889361E-6));
#11571=CARTESIAN_POINT('Ctrl Pts',(0.0920147884934566,1.34020361352282,
4.19020214765608E-6));
#11572=CARTESIAN_POINT('Ctrl Pts',(0.082263696775192,1.33031540618347,-1.43705507633734E-6));
#11573=CARTESIAN_POINT('Ctrl Pts',(0.0732179607829324,1.31975004019149,
-7.24116446069057E-6));
#11574=CARTESIAN_POINT('Ctrl Pts',(0.0614369648181435,1.30598990677343,
-1.48003270644599E-5));
#11575=CARTESIAN_POINT('Ctrl Pts',(0.0509520748529884,1.29120077200215,
-2.24515165560165E-5));
#11576=CARTESIAN_POINT('Ctrl Pts',(0.0418305631051555,1.27560026299671,
-2.64881615939377E-5));
#11577=CARTESIAN_POINT('Ctrl Pts',(0.0329966685655992,1.26049166530727,
-3.03975241584371E-5));
#11578=CARTESIAN_POINT('Ctrl Pts',(0.0254411283904758,1.24462062939249,
-3.09701348507133E-5));
#11579=CARTESIAN_POINT('Ctrl Pts',(0.0192647836588538,1.2281607987719,-2.81763116144976E-5));
#11580=CARTESIAN_POINT('Ctrl Pts',(0.0129258683931997,1.2112677210496,-2.53089508159798E-5));
#11581=CARTESIAN_POINT('Ctrl Pts',(0.00809110271874438,1.19389182855556,
-1.89493195503086E-5));
#11582=CARTESIAN_POINT('Ctrl Pts',(0.00484442764459327,1.17622983835018,
-1.25518552566888E-5));
#11583=CARTESIAN_POINT('Ctrl Pts',(0.00165723550742335,1.1588914367474,
-6.27160009448058E-6));
#11584=CARTESIAN_POINT('Ctrl Pts',(1.90718451428807E-9,1.14127598190669,
-1.51296892603399E-10));
#11585=CARTESIAN_POINT('Ctrl Pts',(2.41777084464267E-17,1.12356026268968,
-3.46944695195361E-18));
#11586=CARTESIAN_POINT('',(10.5166159648474,1.4155315881283,0.));
#11587=CARTESIAN_POINT('Ctrl Pts',(0.276326924564679,1.42224670711126,0.));
#11588=CARTESIAN_POINT('Ctrl Pts',(3.68975660465893,1.68747752195839,0.));
#11589=CARTESIAN_POINT('Ctrl Pts',(7.10318628475318,1.599994843061,0.));
#11590=CARTESIAN_POINT('Ctrl Pts',(10.5166159648474,1.4155315881283,0.));
#11591=CARTESIAN_POINT('',(10.8,1.11638029377732,-5.56631991785941E-17));
#11592=CARTESIAN_POINT('Ctrl Pts',(10.8,1.11638029377732,2.32452945780892E-16));
#11593=CARTESIAN_POINT('Ctrl Pts',(10.7999999994302,1.13421844616111,-9.29296349749781E-12));
#11594=CARTESIAN_POINT('Ctrl Pts',(10.7983603663884,1.15198349698667,-2.38856955364628E-6));
#11595=CARTESIAN_POINT('Ctrl Pts',(10.7951843826221,1.16946861094468,-3.77014304120448E-6));
#11596=CARTESIAN_POINT('Ctrl Pts',(10.7919669771209,1.18718176881198,-5.16973525142236E-6));
#11597=CARTESIAN_POINT('Ctrl Pts',(10.7871724978816,1.20460918321158,-5.4755482503851E-6));
#11598=CARTESIAN_POINT('Ctrl Pts',(10.7808573412527,1.22152732075962,-4.27334038376583E-6));
#11599=CARTESIAN_POINT('Ctrl Pts',(10.7797421066656,1.22451500471617,-4.06103467663179E-6));
#11600=CARTESIAN_POINT('Ctrl Pts',(10.7785793293545,1.22748675045939,-3.81081650224554E-6));
#11601=CARTESIAN_POINT('Ctrl Pts',(10.7773691713543,1.23044124224994,-3.53261416912234E-6));
#11602=CARTESIAN_POINT('Ctrl Pts',(10.7705159051166,1.24717287467681,-1.95712183132163E-6));
#11603=CARTESIAN_POINT('Ctrl Pts',(10.7622076549587,1.26320448426569,8.50150473021234E-7));
#11604=CARTESIAN_POINT('Ctrl Pts',(10.7525236566209,1.27832128496499,1.09915986206012E-6));
#11605=CARTESIAN_POINT('Ctrl Pts',(10.7482509716548,1.28499098118248,1.20902550183604E-6));
#11606=CARTESIAN_POINT('Ctrl Pts',(10.7437098328292,1.29148238441373,7.76315258636623E-7));
#11607=CARTESIAN_POINT('Ctrl Pts',(10.7389041877712,1.29777551763099,-7.54184826032082E-7));
#11608=CARTESIAN_POINT('Ctrl Pts',(10.7310976851069,1.30799836193882,-3.24039694621926E-6));
#11609=CARTESIAN_POINT('Ctrl Pts',(10.7225935645301,1.31769858917671,-8.57388820182801E-6));
#11610=CARTESIAN_POINT('Ctrl Pts',(10.7134588931078,1.3268364513864,-1.41086939541967E-5));
#11611=CARTESIAN_POINT('Ctrl Pts',(10.7004433550849,1.33985653580309,-2.19949628070403E-5));
#11612=CARTESIAN_POINT('Ctrl Pts',(10.6862650266646,1.35162127070648,-3.0022236679635E-5));
#11613=CARTESIAN_POINT('Ctrl Pts',(10.6711476119081,1.36204513612776,-3.40981369893719E-5));
#11614=CARTESIAN_POINT('Ctrl Pts',(10.6560301971515,1.37246900154903,-3.81740372991087E-5));
#11615=CARTESIAN_POINT('Ctrl Pts',(10.6399721826852,1.38155285075117,-3.83332859284948E-5));
#11616=CARTESIAN_POINT('Ctrl Pts',(10.6231652498763,1.38916602817047,-3.45204725343976E-5));
#11617=CARTESIAN_POINT('Ctrl Pts',(10.6063487480974,1.39678354012646,-3.07054883279539E-5));
#11618=CARTESIAN_POINT('Ctrl Pts',(10.5889271210941,1.40286310406803,-2.29928881382306E-5));
#11619=CARTESIAN_POINT('Ctrl Pts',(10.5711041279812,1.40730078588308,-1.53078138731408E-5));
#11620=CARTESIAN_POINT('Ctrl Pts',(10.5532811348684,1.41173846769814,-7.6227396080509E-6));
#11621=CARTESIAN_POINT('Ctrl Pts',(10.5350552605908,1.41453511891929,-9.16729947674095E-11));
#11622=CARTESIAN_POINT('Ctrl Pts',(10.5166159648474,1.4155315881283,2.48932818802672E-16));
#11623=CARTESIAN_POINT('',(10.8,-1.11638029377732,-1.39157997946485E-17));
#11624=CARTESIAN_POINT('',(10.8,1.4,0.));
#11625=CARTESIAN_POINT('',(10.5166159648474,-1.4155315881283,2.77555756156289E-17));
#11626=CARTESIAN_POINT('Ctrl Pts',(10.5166159648474,-1.4155315881283,-1.94289029309402E-16));
#11627=CARTESIAN_POINT('Ctrl Pts',(10.5344251606169,-1.41456917089032,1.72780596414851E-12));
#11628=CARTESIAN_POINT('Ctrl Pts',(10.5520727686739,-1.41197333457428,-2.53403886306205E-6));
#11629=CARTESIAN_POINT('Ctrl Pts',(10.5693578805681,-1.40785843881911,-4.04156906196095E-6));
#11630=CARTESIAN_POINT('Ctrl Pts',(10.5868701251756,-1.40368947182374,-5.56890876087065E-6));
#11631=CARTESIAN_POINT('Ctrl Pts',(10.604011804524,-1.39796079212135,-5.98742339745246E-6));
#11632=CARTESIAN_POINT('Ctrl Pts',(10.6205627760847,-1.39074087128671,-4.81856832951796E-6));
#11633=CARTESIAN_POINT('Ctrl Pts',(10.6234754753687,-1.38947028374636,-4.61286902618664E-6));
#11634=CARTESIAN_POINT('Ctrl Pts',(10.6263698187278,-1.38815339768352,-4.36721670635639E-6));
#11635=CARTESIAN_POINT('Ctrl Pts',(10.629244514885,-1.38679044403738,-4.09122931699412E-6));
#11636=CARTESIAN_POINT('Ctrl Pts',(10.6455827855986,-1.37904412775797,-2.5226612199239E-6));
#11637=CARTESIAN_POINT('Ctrl Pts',(10.6611432679573,-1.36988219838444,3.58605122725343E-7));
#11638=CARTESIAN_POINT('Ctrl Pts',(10.6757157985124,-1.35939560704671,7.40589063327193E-7));
#11639=CARTESIAN_POINT('Ctrl Pts',(10.6821516119741,-1.35476430808026,9.09288478831296E-7));
#11640=CARTESIAN_POINT('Ctrl Pts',(10.6883944859408,-1.34987400891586,5.44816430868337E-7));
#11641=CARTESIAN_POINT('Ctrl Pts',(10.6944246343503,-1.34472976213865,-9.14752338109426E-7));
#11642=CARTESIAN_POINT('Ctrl Pts',(10.7041966733629,-1.33639335368171,-3.28002794718031E-6));
#11643=CARTESIAN_POINT('Ctrl Pts',(10.7134106653983,-1.3273903805878,-8.47259327327479E-6));
#11644=CARTESIAN_POINT('Ctrl Pts',(10.7220307555455,-1.31778973409553,-1.38734771921913E-5));
#11645=CARTESIAN_POINT('Ctrl Pts',(10.7343338492722,-1.3040871333553,-2.15819326638919E-5));
#11646=CARTESIAN_POINT('Ctrl Pts',(10.7453199276401,-1.28929041974124,-2.94555326738194E-5));
#11647=CARTESIAN_POINT('Ctrl Pts',(10.7549158277293,-1.27362793268665,-3.3443536645081E-5));
#11648=CARTESIAN_POINT('Ctrl Pts',(10.7645117278185,-1.25796544563206,-3.74315406163426E-5));
#11649=CARTESIAN_POINT('Ctrl Pts',(10.7727182208071,-1.24143562566754,-3.75750290962259E-5));
#11650=CARTESIAN_POINT('Ctrl Pts',(10.7794153247677,-1.22423716044977,-3.38265125308188E-5));
#11651=CARTESIAN_POINT('Ctrl Pts',(10.7861166764432,-1.20702778690835,-3.00756184258222E-5));
#11652=CARTESIAN_POINT('Ctrl Pts',(10.7912490477072,-1.18929683429644,-2.25107044755726E-5));
#11653=CARTESIAN_POINT('Ctrl Pts',(10.7947196858669,-1.17125359626911,-1.49815203503087E-5));
#11654=CARTESIAN_POINT('Ctrl Pts',(10.7981903240266,-1.15321035824179,-7.45233622504479E-6));
#11655=CARTESIAN_POINT('Ctrl Pts',(10.7999999985278,-1.13485327409571,-1.17780195603766E-10));
#11656=CARTESIAN_POINT('Ctrl Pts',(10.8,-1.11638029377732,-1.38777878078145E-17));
#11657=CARTESIAN_POINT('',(0.276326924564679,-1.42224670711126,-5.55111512312578E-17));
#11658=CARTESIAN_POINT('Ctrl Pts',(10.5166159648474,-1.4155315881283,0.));
#11659=CARTESIAN_POINT('Ctrl Pts',(7.10318628475318,-1.599994843061,0.));
#11660=CARTESIAN_POINT('Ctrl Pts',(3.68975660465893,-1.68747752195839,0.));
#11661=CARTESIAN_POINT('Ctrl Pts',(0.276326924564679,-1.42224670711126,
0.));
#11662=CARTESIAN_POINT('',(-7.25311916552711E-19,-1.12356026268968,1.39157997946485E-17));
#11663=CARTESIAN_POINT('Ctrl Pts',(1.80411241501588E-16,-1.12356026268968,
-1.53523027623947E-16));
#11664=CARTESIAN_POINT('Ctrl Pts',(7.41078168374529E-10,-1.14141522098415,
-1.3067981184062E-11));
#11665=CARTESIAN_POINT('Ctrl Pts',(0.00163694718329378,-1.15920272117896,
-1.78823819589733E-6));
#11666=CARTESIAN_POINT('Ctrl Pts',(0.00481087395297265,-1.17671209893291,
-2.3181425555783E-6));
#11667=CARTESIAN_POINT('Ctrl Pts',(0.00802138847203439,-1.19442331774104,
-2.85415543927884E-6));
#11668=CARTESIAN_POINT('Ctrl Pts',(0.0128049030182357,-1.21185152247087,
-2.04128886843626E-6));
#11669=CARTESIAN_POINT('Ctrl Pts',(0.0191087770915565,-1.22877027194193,
1.71240493184593E-7));
#11670=CARTESIAN_POINT('Ctrl Pts',(0.0202201941454154,-1.23175316571065,
5.613248819379E-7));
#11671=CARTESIAN_POINT('Ctrl Pts',(0.0213789882593307,-1.23472016785247,
9.85829603970989E-7));
#11672=CARTESIAN_POINT('Ctrl Pts',(0.0225850188675993,-1.23766995297306,
1.43287414332239E-6));
#11673=CARTESIAN_POINT('Ctrl Pts',(0.0294291562303479,-1.25440977235863,
3.96981990042924E-6));
#11674=CARTESIAN_POINT('Ctrl Pts',(0.0377300686697735,-1.27044838970616,
7.55798501181421E-6));
#11675=CARTESIAN_POINT('Ctrl Pts',(0.0474121614036163,-1.28556782977674,
8.05058320302158E-6));
#11676=CARTESIAN_POINT('Ctrl Pts',(0.0511425121829324,-1.29139310088294,
8.24037316857697E-6));
#11677=CARTESIAN_POINT('Ctrl Pts',(0.0550784035723718,-1.29708174651376,
7.93435480917585E-6));
#11678=CARTESIAN_POINT('Ctrl Pts',(0.0592173503759339,-1.30262033374061,
6.74858081742264E-6));
#11679=CARTESIAN_POINT('Ctrl Pts',(0.0675201807396794,-1.31373087764993,
4.36988865960166E-6));
#11680=CARTESIAN_POINT('Ctrl Pts',(0.0766394565597649,-1.32423847988766,
-1.46587651676554E-6));
#11681=CARTESIAN_POINT('Ctrl Pts',(0.0864911062490747,-1.33409287340636,
-7.46705500292641E-6));
#11682=CARTESIAN_POINT('Ctrl Pts',(0.0992988409846585,-1.34690417528452,
-1.52689465211603E-5));
#11683=CARTESIAN_POINT('Ctrl Pts',(0.113232871116931,-1.35850278376499,
-2.31308069859054E-5));
#11684=CARTESIAN_POINT('Ctrl Pts',(0.128081622025101,-1.36880445085772,
-2.72849174168177E-5));
#11685=CARTESIAN_POINT('Ctrl Pts',(0.142447925282442,-1.37877140864598,
-3.13040575171566E-5));
#11686=CARTESIAN_POINT('Ctrl Pts',(0.157671864768995,-1.38752483454192,
-3.1899138628041E-5));
#11687=CARTESIAN_POINT('Ctrl Pts',(0.173588691395025,-1.39495074934422,
-2.90326641197332E-5));
#11688=CARTESIAN_POINT('Ctrl Pts',(0.189936400238013,-1.40257769006131,
-2.60885916756054E-5));
#11689=CARTESIAN_POINT('Ctrl Pts',(0.206881864105471,-1.40874232120582,
-1.95409011442111E-5));
#11690=CARTESIAN_POINT('Ctrl Pts',(0.22423558959196,-1.41334558507228,-1.29462590315495E-5));
#11691=CARTESIAN_POINT('Ctrl Pts',(0.241260467995769,-1.4178616186841,-6.47658310103417E-6));
#11692=CARTESIAN_POINT('Ctrl Pts',(0.258679581942429,-1.42087546890512,
-1.12101563992788E-10));
#11693=CARTESIAN_POINT('Ctrl Pts',(0.27632692456468,-1.42224670711126,1.05818132034585E-16));
#11694=CARTESIAN_POINT('',(0.,-1.4,0.));
#11695=CARTESIAN_POINT('',(0.292382661757373,-1.22257596919059,0.));
#11696=CARTESIAN_POINT('Ctrl Pts',(0.200274469199584,-1.12301388185427,
-2.68882138776405E-17));
#11697=CARTESIAN_POINT('Ctrl Pts',(0.200274469314753,-1.13095194822878,
-2.85686379674833E-12));
#11698=CARTESIAN_POINT('Ctrl Pts',(0.201244085522878,-1.13884856843413,
-1.08105759021766E-6));
#11699=CARTESIAN_POINT('Ctrl Pts',(0.203110344361254,-1.14653799330522,
-1.10782444979703E-6));
#11700=CARTESIAN_POINT('Ctrl Pts',(0.204308287281872,-1.15147379958167,
-1.12500597321754E-6));
#11701=CARTESIAN_POINT('Ctrl Pts',(0.205876831658669,-1.15632444796435,
-7.573778542164E-7));
#11702=CARTESIAN_POINT('Ctrl Pts',(0.207807574899602,-1.16104329283393,
-1.57887042599725E-7));
#11703=CARTESIAN_POINT('Ctrl Pts',(0.21096922807971,-1.1687705506961,8.23798139982571E-7));
#11704=CARTESIAN_POINT('Ctrl Pts',(0.215060220496011,-1.17605061753432,
2.67511715935828E-6));
#11705=CARTESIAN_POINT('Ctrl Pts',(0.220020901709485,-1.18268777995331,
1.20301732358232E-6));
#11706=CARTESIAN_POINT('Ctrl Pts',(0.222788929945646,-1.18639127392786,
3.81595076007225E-7));
#11707=CARTESIAN_POINT('Ctrl Pts',(0.225828882930032,-1.18989419630164,
-1.55522758636672E-6));
#11708=CARTESIAN_POINT('Ctrl Pts',(0.229112809647272,-1.19317965616817,
-3.52099818518546E-6));
#11709=CARTESIAN_POINT('Ctrl Pts',(0.234731790749985,-1.1988012605745,-6.88454091865859E-6));
#11710=CARTESIAN_POINT('Ctrl Pts',(0.240999377733319,-1.20372479786492,
-1.00686973618824E-5));
#11711=CARTESIAN_POINT('Ctrl Pts',(0.247759525934523,-1.2078808899968,-1.07387199666626E-5));
#11712=CARTESIAN_POINT('Ctrl Pts',(0.251104201987095,-1.20993717358883,
-1.10702228411842E-5));
#11713=CARTESIAN_POINT('Ctrl Pts',(0.254570062984725,-1.21180502729412,
-1.08478245319173E-5));
#11714=CARTESIAN_POINT('Ctrl Pts',(0.258140701417296,-1.21347208138814,
-1.01264154182862E-5));
#11715=CARTESIAN_POINT('Ctrl Pts',(0.265309933881728,-1.21681924144269,
-8.67794906268977E-6));
#11716=CARTESIAN_POINT('Ctrl Pts',(0.27282354441991,-1.21932394229889,-5.03816435877804E-6));
#11717=CARTESIAN_POINT('Ctrl Pts',(0.280540402387729,-1.22090470300999,
-2.38011023443526E-6));
#11718=CARTESIAN_POINT('Ctrl Pts',(0.284441227387562,-1.22170376798259,
-1.03647996128718E-6));
#11719=CARTESIAN_POINT('Ctrl Pts',(0.288394358015454,-1.22226603782358,
-8.41267709508591E-12));
#11720=CARTESIAN_POINT('Ctrl Pts',(0.292382661757373,-1.22257596919059,
3.10081821330854E-17));
#11721=CARTESIAN_POINT('',(0.9,-1.266106713614,0.));
#11722=CARTESIAN_POINT('Ctrl Pts',(0.29238266175737,-1.22257596919059,3.4274341177698E-16));
#11723=CARTESIAN_POINT('Ctrl Pts',(0.494894519961671,-1.23831317320793,
3.6654050078524E-12));
#11724=CARTESIAN_POINT('Ctrl Pts',(0.697432753591781,-1.25280566766171,
-2.10377631034678E-8));
#11725=CARTESIAN_POINT('Ctrl Pts',(0.900000000000002,-1.266106713614,4.80511808774455E-17));
#11726=CARTESIAN_POINT('',(0.9,1.34328341716202,0.));
#11727=CARTESIAN_POINT('',(3.5,-1.37552980833516,0.));
#11728=CARTESIAN_POINT('Ctrl Pts',(1.10000000028363,-1.27885335028943,-5.13283219638443E-11));
#11729=CARTESIAN_POINT('Ctrl Pts',(1.8994825293422,-1.32827224294784,2.51289069808066E-7));
#11730=CARTESIAN_POINT('Ctrl Pts',(2.69943073922525,-1.35940904940056,2.35357980118634E-7));
#11731=CARTESIAN_POINT('Ctrl Pts',(3.50000000097418,-1.37552980835478,8.59034485311056E-16));
#11732=CARTESIAN_POINT('',(3.5,1.44777777777778,0.));
#11733=CARTESIAN_POINT('',(7.1,-1.35793097395724,0.));
#11734=CARTESIAN_POINT('Ctrl Pts',(3.700000000362,-1.379246395385,-6.25385501848083E-12));
#11735=CARTESIAN_POINT('Ctrl Pts',(4.26467016042339,-1.38886773733237,1.63880713394601E-8));
#11736=CARTESIAN_POINT('Ctrl Pts',(4.82965558050887,-1.39115503781354,-4.12727732537403E-8));
#11737=CARTESIAN_POINT('Ctrl Pts',(5.39500817395676,-1.38725486475042,-3.97626883737645E-8));
#11738=CARTESIAN_POINT('Ctrl Pts',(5.96336684492344,-1.38333395379258,-3.82445741104923E-8));
#11739=CARTESIAN_POINT('Ctrl Pts',(6.53173538886785,-1.37316170188981,3.71969681223073E-9));
#11740=CARTESIAN_POINT('Ctrl Pts',(7.1000000000396,-1.35793097389613,-4.88946831112289E-12));
#11741=CARTESIAN_POINT('',(7.1,1.42555555555556,0.));
#11742=CARTESIAN_POINT('',(10.2,-1.23178301601145,0.));
#11743=CARTESIAN_POINT('',(10.5052647440597,-1.21555035534119,0.));
#11744=CARTESIAN_POINT('Ctrl Pts',(10.2,-1.23178301601145,-4.56855690431079E-17));
#11745=CARTESIAN_POINT('Ctrl Pts',(10.3017652114452,-1.22646242153193,-6.28718440835499E-11));
#11746=CARTESIAN_POINT('Ctrl Pts',(10.4035203469111,-1.22104923788321,1.43982679105611E-13));
#11747=CARTESIAN_POINT('Ctrl Pts',(10.5052647440597,-1.21555035534119,6.44897004721534E-17));
#11748=CARTESIAN_POINT('',(10.5997255308004,-1.11583328740478,1.38777878078145E-17));
#11749=CARTESIAN_POINT('Ctrl Pts',(10.5052647440597,-1.21555035534119,-1.86482773667507E-17));
#11750=CARTESIAN_POINT('Ctrl Pts',(10.5131888530666,-1.21512208850275,-5.60416335832109E-13));
#11751=CARTESIAN_POINT('Ctrl Pts',(10.5210180054001,-1.21372544600509,-1.35972994235015E-6));
#11752=CARTESIAN_POINT('Ctrl Pts',(10.5285917824072,-1.2114444991589,-1.66070161277884E-6));
#11753=CARTESIAN_POINT('Ctrl Pts',(10.5334522234388,-1.20998071066451,-1.8538489757029E-6));
#11754=CARTESIAN_POINT('Ctrl Pts',(10.538207639053,-1.20815156029678,-1.66445033219183E-6));
#11755=CARTESIAN_POINT('Ctrl Pts',(10.542812250732,-1.20596855068549,-1.19054254011085E-6));
#11756=CARTESIAN_POINT('Ctrl Pts',(10.5499808226381,-1.20256998801374,-4.52751316616249E-7));
#11757=CARTESIAN_POINT('Ctrl Pts',(10.5567010840309,-1.19835579238971,1.16775294480959E-6));
#11758=CARTESIAN_POINT('Ctrl Pts',(10.5628099082467,-1.1933896765605,3.12218506849373E-7));
#11759=CARTESIAN_POINT('Ctrl Pts',(10.563392699667,-1.1929159013142,2.30599178383296E-7));
#11760=CARTESIAN_POINT('Ctrl Pts',(10.563969906567,-1.19243524850296,1.23643260424227E-7));
#11761=CARTESIAN_POINT('Ctrl Pts',(10.5645413730323,-1.19194775268147,-1.33988689923433E-8));
#11762=CARTESIAN_POINT('Ctrl Pts',(10.5677990734116,-1.18916873515523,-7.94620907596477E-7));
#11763=CARTESIAN_POINT('Ctrl Pts',(10.5708705204042,-1.18616755700159,-2.52696578471864E-6));
#11764=CARTESIAN_POINT('Ctrl Pts',(10.5737438185805,-1.18296717200411,-4.3349897000341E-6));
#11765=CARTESIAN_POINT('Ctrl Pts',(10.579054042416,-1.17705244973962,-7.67644996655303E-6));
#11766=CARTESIAN_POINT('Ctrl Pts',(10.5836289246435,-1.17052745137283,-1.0999028846932E-5));
#11767=CARTESIAN_POINT('Ctrl Pts',(10.5874112735695,-1.16355342251842,-1.18035167459916E-5));
#11768=CARTESIAN_POINT('Ctrl Pts',(10.5894705469099,-1.15975646143,-1.22415145393192E-5));
#11769=CARTESIAN_POINT('Ctrl Pts',(10.5912942421259,-1.15582570378367,-1.20038889321768E-5));
#11770=CARTESIAN_POINT('Ctrl Pts',(10.5928674986933,-1.15178403025788,-1.11465830745351E-5));
#11771=CARTESIAN_POINT('Ctrl Pts',(10.5957384082276,-1.14440870489779,-9.58215448007377E-6));
#11772=CARTESIAN_POINT('Ctrl Pts',(10.5977463817932,-1.13674651935037,-5.80208140981121E-6));
#11773=CARTESIAN_POINT('Ctrl Pts',(10.5988207707371,-1.12894377506163,-2.8960211281105E-6));
#11774=CARTESIAN_POINT('Ctrl Pts',(10.5994175893465,-1.12460938291963,-1.28171667533415E-6));
#11775=CARTESIAN_POINT('Ctrl Pts',(10.5997255306822,-1.12023121224821,-9.4020583932734E-12));
#11776=CARTESIAN_POINT('Ctrl Pts',(10.5997255308004,-1.11583328740478,-9.97465998686664E-18));
#11777=CARTESIAN_POINT('',(10.5997255308004,1.11583328740478,0.));
#11778=CARTESIAN_POINT('',(10.5997255308004,0.7,0.));
#11779=CARTESIAN_POINT('',(10.5052647440597,1.21555035534119,0.));
#11780=CARTESIAN_POINT('Ctrl Pts',(10.5997255308004,1.11583328740478,8.8037216405823E-17));
#11781=CARTESIAN_POINT('Ctrl Pts',(10.5997255307124,1.12376989384288,-2.22024716398596E-12));
#11782=CARTESIAN_POINT('Ctrl Pts',(10.5987536115518,1.13166401228391,-1.27532141444775E-6));
#11783=CARTESIAN_POINT('Ctrl Pts',(10.5968849989732,1.13935090273995,-1.5236651967046E-6));
#11784=CARTESIAN_POINT('Ctrl Pts',(10.5956849616024,1.14428748291596,-1.68315348385219E-6));
#11785=CARTESIAN_POINT('Ctrl Pts',(10.5941139374364,1.14913880701507,-1.46899737395989E-6));
#11786=CARTESIAN_POINT('Ctrl Pts',(10.5921809408638,1.1538584293407,-9.90118991603547E-7));
#11787=CARTESIAN_POINT('Ctrl Pts',(10.5891742477341,1.16119959911942,-2.45244239835432E-7));
#11788=CARTESIAN_POINT('Ctrl Pts',(10.5853292249979,1.16813727090899,1.33309554558619E-6));
#11789=CARTESIAN_POINT('Ctrl Pts',(10.5807005079991,1.17450509276749,4.08358240744415E-7));
#11790=CARTESIAN_POINT('Ctrl Pts',(10.5802604812716,1.17511044665166,3.20448539159982E-7));
#11791=CARTESIAN_POINT('Ctrl Pts',(10.5798133373602,1.17571063303672,2.07176952714776E-7));
#11792=CARTESIAN_POINT('Ctrl Pts',(10.5793591019426,1.17630549598644,6.38823567561716E-8));
#11793=CARTESIAN_POINT('Ctrl Pts',(10.5767566952267,1.17971358631841,-7.57081408668461E-7));
#11794=CARTESIAN_POINT('Ctrl Pts',(10.5739217504488,1.18294722379721,-2.53660858190298E-6));
#11795=CARTESIAN_POINT('Ctrl Pts',(10.570876618072,1.18599321478588,-4.38998728286835E-6));
#11796=CARTESIAN_POINT('Ctrl Pts',(10.5652565693637,1.19161484813492,-7.81055403847458E-6));
#11797=CARTESIAN_POINT('Ctrl Pts',(10.5589874561388,1.19653507038546,-1.11999964534866E-5));
#11798=CARTESIAN_POINT('Ctrl Pts',(10.5522271124844,1.20068789486255,-1.20263298844839E-5));
#11799=CARTESIAN_POINT('Ctrl Pts',(10.5485500617744,1.20294667739977,-1.24757848359648E-5));
#11800=CARTESIAN_POINT('Ctrl Pts',(10.5447269560479,1.20497781184918,-1.22374322375965E-5));
#11801=CARTESIAN_POINT('Ctrl Pts',(10.5407797717187,1.20676523914267,-1.13674773191707E-5));
#11802=CARTESIAN_POINT('Ctrl Pts',(10.5335711832013,1.210029547771,-9.77871264224002E-6));
#11803=CARTESIAN_POINT('Ctrl Pts',(10.5260296312848,1.21244761587922,-5.9245235663186E-6));
#11804=CARTESIAN_POINT('Ctrl Pts',(10.5182973307397,1.21394093281975,-2.95733858081469E-6));
#11805=CARTESIAN_POINT('Ctrl Pts',(10.514004731837,1.21476995008607,-1.31010113336685E-6));
#11806=CARTESIAN_POINT('Ctrl Pts',(10.5096528988527,1.21531319279956,-7.28166367327128E-12));
#11807=CARTESIAN_POINT('Ctrl Pts',(10.5052647440597,1.21555035534119,-3.31765864780564E-17));
#11808=CARTESIAN_POINT('',(10.2,1.23178301601145,0.));
#11809=CARTESIAN_POINT('Ctrl Pts',(10.5052647440597,1.21555035534119,1.20285454773689E-16));
#11810=CARTESIAN_POINT('Ctrl Pts',(10.4035203468995,1.22104923788384,1.44021921739714E-13));
#11811=CARTESIAN_POINT('Ctrl Pts',(10.3017652114309,1.22646242153268,-6.28696045710378E-11));
#11812=CARTESIAN_POINT('Ctrl Pts',(10.2,1.23178301601145,1.23125603768043E-16));
#11813=CARTESIAN_POINT('',(10.2,-1.30754691548544,0.));
#11814=CARTESIAN_POINT('Origin',(8.8,0.,0.));
#11815=CARTESIAN_POINT('',(8.4,-4.89858719658942E-17,0.));
#11816=CARTESIAN_POINT('Origin',(2.,0.,0.));
#11817=CARTESIAN_POINT('',(1.6,-4.89858719658941E-17,0.7));
#11818=CARTESIAN_POINT('Origin',(2.,0.,0.7));
#11819=CARTESIAN_POINT('',(1.6,-4.89858719658941E-17,0.));
#11820=CARTESIAN_POINT('Origin',(10.2,-1.30754691548544,0.));
#11821=CARTESIAN_POINT('',(10.1999999975107,-1.19856231453552,0.605472757505173));
#11822=CARTESIAN_POINT('Ctrl Pts',(10.2,-1.23178301601145,0.));
#11823=CARTESIAN_POINT('Ctrl Pts',(10.2,-1.22625045235593,0.100869147801815));
#11824=CARTESIAN_POINT('Ctrl Pts',(10.2,-1.22071692450357,0.201739022585575));
#11825=CARTESIAN_POINT('Ctrl Pts',(10.2,-1.2096433936729,0.403562754186249));
#11826=CARTESIAN_POINT('Ctrl Pts',(10.1999999975107,-1.20410330368611,0.50451817268257));
#11827=CARTESIAN_POINT('Ctrl Pts',(10.1999999975107,-1.19856231453552,0.605472757505173));
#11828=CARTESIAN_POINT('',(10.1999999975107,1.19856231453552,0.605472757505173));
#11829=CARTESIAN_POINT('Ctrl Pts',(10.1999999975107,1.19856231453552,0.605472757505173));
#11830=CARTESIAN_POINT('Ctrl Pts',(10.1999999975107,1.20410418062036,0.504502195294633));
#11831=CARTESIAN_POINT('Ctrl Pts',(10.2,1.20964514726505,0.403530798997214));
#11832=CARTESIAN_POINT('Ctrl Pts',(10.2,1.22071867750565,0.201707067365009));
#11833=CARTESIAN_POINT('Ctrl Pts',(10.2,1.22625132869937,0.100853170395858));
#11834=CARTESIAN_POINT('Ctrl Pts',(10.2,1.23178301601145,0.));
#11835=CARTESIAN_POINT('',(10.1999999980542,1.09857320530976,0.7));
#11836=CARTESIAN_POINT('Ctrl Pts',(10.1999999999973,1.09857320510493,0.7));
#11837=CARTESIAN_POINT('Ctrl Pts',(10.2000000008642,1.10649088744708,0.699999999248278));
#11838=CARTESIAN_POINT('Ctrl Pts',(10.1999989363772,1.11434529358656,0.699006164779054));
#11839=CARTESIAN_POINT('Ctrl Pts',(10.1999980093114,1.12199598895487,0.697118997523365));
#11840=CARTESIAN_POINT('Ctrl Pts',(10.1999974900707,1.12628106973794,0.696062013320951));
#11841=CARTESIAN_POINT('Ctrl Pts',(10.1999970168623,1.13050229860485,0.694723760583242));
#11842=CARTESIAN_POINT('Ctrl Pts',(10.199996713894,1.13463332887353,0.693115046692397));
#11843=CARTESIAN_POINT('Ctrl Pts',(10.1999961690675,1.14206214329588,0.690222103243312));
#11844=CARTESIAN_POINT('Ctrl Pts',(10.1999962772589,1.14911941279843,0.686488866209959));
#11845=CARTESIAN_POINT('Ctrl Pts',(10.1999969599022,1.15565885618684,0.681996408643444));
#11846=CARTESIAN_POINT('Ctrl Pts',(10.1999973343062,1.15924549304116,0.679532465931891));
#11847=CARTESIAN_POINT('Ctrl Pts',(10.1999978674396,1.16267609380848,0.676839263748528));
#11848=CARTESIAN_POINT('Ctrl Pts',(10.1999983417863,1.16592263776853,0.673924718551186));
#11849=CARTESIAN_POINT('Ctrl Pts',(10.199998806773,1.16910511991263,0.671067684066867));
#11850=CARTESIAN_POINT('Ctrl Pts',(10.1999992207276,1.17209141256199,0.668015240668471));
#11851=CARTESIAN_POINT('Ctrl Pts',(10.1999992206607,1.17485880184773,0.664778864469812));
#11852=CARTESIAN_POINT('Ctrl Pts',(10.1999992205369,1.17997899231675,0.658790960038769));
#11853=CARTESIAN_POINT('Ctrl Pts',(10.1999979581638,1.18435276586188,0.652174799271591));
#11854=CARTESIAN_POINT('Ctrl Pts',(10.1999975326045,1.18791964688485,0.645095405674036));
#11855=CARTESIAN_POINT('Ctrl Pts',(10.1999974898604,1.18827791229431,0.644384335742179));
#11856=CARTESIAN_POINT('Ctrl Pts',(10.1999974535047,1.18862799840101,0.643668573506599));
#11857=CARTESIAN_POINT('Ctrl Pts',(10.1999974242393,1.18896981696374,0.64294827577739));
#11858=CARTESIAN_POINT('Ctrl Pts',(10.1999971329942,1.1923715530028,0.635779961907205));
#11859=CARTESIAN_POINT('Ctrl Pts',(10.1999977790614,1.19491900203126,0.628247233077589));
#11860=CARTESIAN_POINT('Ctrl Pts',(10.1999987199397,1.19655829940385,0.620518158911201));
#11861=CARTESIAN_POINT('Ctrl Pts',(10.1999993222661,1.19760773597399,0.615570201805241));
#11862=CARTESIAN_POINT('Ctrl Pts',(10.2,1.19828413277105,0.610541112135461));
#11863=CARTESIAN_POINT('Ctrl Pts',(10.2,1.19856231427281,0.60547275750556));
#11864=CARTESIAN_POINT('',(10.2,-1.09857320510402,0.7));
#11865=CARTESIAN_POINT('',(10.2,-0.653773457742722,0.7));
#11866=CARTESIAN_POINT('Ctrl Pts',(10.2,-1.19856231427281,0.60547275750556));
#11867=CARTESIAN_POINT('Ctrl Pts',(10.2,-1.19812809376428,0.613384079828744));
#11868=CARTESIAN_POINT('Ctrl Pts',(10.1999984889428,-1.1967261327477,0.621202329970501));
#11869=CARTESIAN_POINT('Ctrl Pts',(10.1999978161146,-1.19444079525024,0.628767398200536));
#11870=CARTESIAN_POINT('Ctrl Pts',(10.1999974438306,-1.19317629038787,0.632953241898348));
#11871=CARTESIAN_POINT('Ctrl Pts',(10.1999972759003,-1.19164034846853,0.637061602680377));
#11872=CARTESIAN_POINT('Ctrl Pts',(10.1999973648938,-1.18984073583679,0.641063423920242));
#11873=CARTESIAN_POINT('Ctrl Pts',(10.1999975257516,-1.18658789218766,0.648296813248274));
#11874=CARTESIAN_POINT('Ctrl Pts',(10.1999986492083,-1.18251199594868,0.655103972585077));
#11875=CARTESIAN_POINT('Ctrl Pts',(10.1999990866637,-1.1776776067306,0.66132208754656));
#11876=CARTESIAN_POINT('Ctrl Pts',(10.1999991692372,-1.17676507450965,0.662495809810115));
#11877=CARTESIAN_POINT('Ctrl Pts',(10.1999992204458,-1.17582538639523,0.663648473741297));
#11878=CARTESIAN_POINT('Ctrl Pts',(10.1999992199672,-1.17485880188435,0.664778864469789));
#11879=CARTESIAN_POINT('Ctrl Pts',(10.1999992190419,-1.17299032792757,0.666963987046661));
#11880=CARTESIAN_POINT('Ctrl Pts',(10.1999990265713,-1.17102137903347,0.669065925022507));
#11881=CARTESIAN_POINT('Ctrl Pts',(10.1999987631451,-1.16895889720817,0.671081139337088));
#11882=CARTESIAN_POINT('Ctrl Pts',(10.1999980371048,-1.16327440276409,0.676635357771578));
#11883=CARTESIAN_POINT('Ctrl Pts',(10.1999968952367,-1.15694629605269,0.681471105251756));
#11884=CARTESIAN_POINT('Ctrl Pts',(10.1999965193249,-1.15013861030111,0.685534582868085));
#11885=CARTESIAN_POINT('Ctrl Pts',(10.1999962798276,-1.14580136285465,0.688123466749966));
#11886=CARTESIAN_POINT('Ctrl Pts',(10.1999963003895,-1.14126848503633,0.690398200126003));
#11887=CARTESIAN_POINT('Ctrl Pts',(10.1999965837416,-1.13657664085124,0.692335536714198));
#11888=CARTESIAN_POINT('Ctrl Pts',(10.199997026059,-1.12925259320479,0.695359751696499));
#11889=CARTESIAN_POINT('Ctrl Pts',(10.1999981114625,-1.12162598460505,0.697529439192009));
#11890=CARTESIAN_POINT('Ctrl Pts',(10.1999989867727,-1.11384404680861,0.698775198878229));
#11891=CARTESIAN_POINT('Ctrl Pts',(10.1999995533653,-1.10880676031141,0.699581585232154));
#11892=CARTESIAN_POINT('Ctrl Pts',(10.200000000559,-1.10370379302489,0.699999999512891));
#11893=CARTESIAN_POINT('Ctrl Pts',(10.1999999999973,-1.09857320510493,0.7));
#11894=CARTESIAN_POINT('Ctrl Pts',(10.0273290644374,-1.24073895154929,-0.000342977371441382));
#11895=CARTESIAN_POINT('Ctrl Pts',(10.0182194939277,-1.2301570933055,0.201590462913323));
#11896=CARTESIAN_POINT('Ctrl Pts',(10.0091098064739,-1.21957524432673,0.403523898419685));
#11897=CARTESIAN_POINT('Ctrl Pts',(10.,-1.20899340483173,0.605457329065658));
#11898=CARTESIAN_POINT('Ctrl Pts',(9.11786336174441,-1.287320026752,-0.000205293215301774));
#11899=CARTESIAN_POINT('Ctrl Pts',(9.11054075262461,-1.27673792859995,0.201728409731728));
#11900=CARTESIAN_POINT('Ctrl Pts',(9.10321803982027,-1.2661558351744,0.403662109352091));
#11901=CARTESIAN_POINT('Ctrl Pts',(9.09589522044064,-1.25557375159922,0.605595805683776));
#11902=CARTESIAN_POINT('Ctrl Pts',(8.20875307681921,-1.32613868191631,-8.19769783003664E-5));
#11903=CARTESIAN_POINT('Ctrl Pts',(8.20321812688803,-1.31555630757271,0.201851960079368));
#11904=CARTESIAN_POINT('Ctrl Pts',(8.19768309032111,-1.30497393555236,0.403785895133155));
#11905=CARTESIAN_POINT('Ctrl Pts',(8.19214796413157,-1.29439157095064,0.605719828258773));
#11906=CARTESIAN_POINT('Ctrl Pts',(7.29999999999999,-1.35236351479115,1.04083408558608E-17));
#11907=CARTESIAN_POINT('Ctrl Pts',(7.29625341766944,-1.34178092325774,0.201934092022114));
#11908=CARTESIAN_POINT('Ctrl Pts',(7.2925067690755,-1.33119833465137,0.403868182971915));
#11909=CARTESIAN_POINT('Ctrl Pts',(7.28876005303739,-1.32061574904145,0.605802272831199));
#11910=CARTESIAN_POINT('Ctrl Pts',(7.29999999953094,-1.32031613471704,0.605285370449856));
#11911=CARTESIAN_POINT('Ctrl Pts',(8.20058408060299,-1.29406305600824,0.605326635812744));
#11912=CARTESIAN_POINT('Ctrl Pts',(9.10058974048747,-1.25534320916473,0.605388449123016));
#11913=CARTESIAN_POINT('Ctrl Pts',(9.99999999968202,-1.20899340489109,0.605457329065633));
#11914=CARTESIAN_POINT('Ctrl Pts',(10.5052670937641,-1.21555282972197,-4.72190879230918E-5));
#11915=CARTESIAN_POINT('Ctrl Pts',(10.4952228315222,-1.20497561405085,0.201799837144789));
#11916=CARTESIAN_POINT('Ctrl Pts',(10.4851784461209,-1.19439840869387,0.403646887802288));
#11917=CARTESIAN_POINT('Ctrl Pts',(10.4751339353761,-1.18382121389426,0.605493932788863));
#11918=CARTESIAN_POINT('Ctrl Pts',(10.4035069533234,-1.22105168617584,-3.13467776074076E-5));
#11919=CARTESIAN_POINT('Ctrl Pts',(10.3936624949941,-1.21047444506522,0.201815739766394));
#11920=CARTESIAN_POINT('Ctrl Pts',(10.3838179147697,-1.19989721405033,0.403662820908308));
#11921=CARTESIAN_POINT('Ctrl Pts',(10.3739732104882,-1.18931999337004,0.605509896555428));
#11922=CARTESIAN_POINT('Ctrl Pts',(10.3017512542637,-1.22646400658821,-1.55943981238903E-5));
#11923=CARTESIAN_POINT('Ctrl Pts',(10.2921066085356,-1.21588673949083,0.201831522212972));
#11924=CARTESIAN_POINT('Ctrl Pts',(10.2824618422276,-1.20530948226626,0.403678633593635));
#11925=CARTESIAN_POINT('Ctrl Pts',(10.2728169532007,-1.19473223514815,0.605525739654126));
#11926=CARTESIAN_POINT('Ctrl Pts',(10.2,-1.23178301601145,-4.5102810375397E-17));
#11927=CARTESIAN_POINT('Ctrl Pts',(10.1905551755811,-1.22120572247414,0.20184714636246));
#11928=CARTESIAN_POINT('Ctrl Pts',(10.1811102319487,-1.21062843858304,0.403694287664275));
#11929=CARTESIAN_POINT('Ctrl Pts',(10.1716651669877,-1.20005116456574,0.605541423818621));
#11930=CARTESIAN_POINT('',(10.4735630903435,-1.18390659316268,0.605494180667944));
#11931=CARTESIAN_POINT('Ctrl Pts',(10.1999999975038,-1.19856231440453,0.605472757505366));
#11932=CARTESIAN_POINT('Ctrl Pts',(10.2911933328565,-1.19375025772558,0.605479840815741));
#11933=CARTESIAN_POINT('Ctrl Pts',(10.3823809652617,-1.18886335120032,0.605486986548286));
#11934=CARTESIAN_POINT('Ctrl Pts',(10.4735630903435,-1.18390659316268,0.605494180667944));
#11935=CARTESIAN_POINT('Ctrl Pts',(10.4735630903435,-1.18390659316268,0.605494180667945));
#11936=CARTESIAN_POINT('Ctrl Pts',(10.4841302498201,-1.19445434834508,0.403662775875149));
#11937=CARTESIAN_POINT('Ctrl Pts',(10.4946974680575,-1.20500226999407,0.201831382381129));
#11938=CARTESIAN_POINT('Ctrl Pts',(10.5052647440597,-1.21555035534119,-6.86299975183324E-17));
#11939=CARTESIAN_POINT('Ctrl Pts',(10.,-1.10900986674273,0.7));
#11940=CARTESIAN_POINT('Ctrl Pts',(9.09944331332257,-1.15544418981837,0.7));
#11941=CARTESIAN_POINT('Ctrl Pts',(8.1984670949788,-1.19422430779862,0.7));
#11942=CARTESIAN_POINT('Ctrl Pts',(7.29709043526679,-1.22049830417059,0.7));
#11943=CARTESIAN_POINT('Ctrl Pts',(10.0014871213396,-1.13785139984992,0.7));
#11944=CARTESIAN_POINT('Ctrl Pts',(9.10076698492608,-1.18430758604571,0.700000491839571));
#11945=CARTESIAN_POINT('Ctrl Pts',(8.19957769811723,-1.22310890030201,0.699999704549177));
#11946=CARTESIAN_POINT('Ctrl Pts',(7.29793284700475,-1.24939875264889,0.7));
#11947=CARTESIAN_POINT('Ctrl Pts',(10.0040646682326,-1.18784086746588,0.676686753673613));
#11948=CARTESIAN_POINT('Ctrl Pts',(9.10306300621911,-1.23433322993607,0.676664155483858));
#11949=CARTESIAN_POINT('Ctrl Pts',(8.20149954052229,-1.27317186922949,0.676644146017133));
#11950=CARTESIAN_POINT('Ctrl Pts',(7.29939288958795,-1.29948813715084,0.676630595533454));
#11951=CARTESIAN_POINT('Ctrl Pts',(10.0050807923581,-1.20754778500352,0.627085325222079));
#11952=CARTESIAN_POINT('Ctrl Pts',(9.10396596140607,-1.25402923300358,0.627026849623412));
#11953=CARTESIAN_POINT('Ctrl Pts',(8.20225661204673,-1.29285896783792,0.626974637782525));
#11954=CARTESIAN_POINT('Ctrl Pts',(7.29996660609514,-1.31917051289423,0.626939603849942));
#11955=CARTESIAN_POINT('Ctrl Pts',(10.0051416645797,-1.20872835322339,0.605457722909465));
#11956=CARTESIAN_POINT('Ctrl Pts',(9.1040197884667,-1.25519559703033,0.605388684776982));
#11957=CARTESIAN_POINT('Ctrl Pts',(8.20230020786566,-1.29401302889245,0.605326714446839));
#11958=CARTESIAN_POINT('Ctrl Pts',(7.29999999953094,-1.32031613471704,0.605285370449856));
#11959=CARTESIAN_POINT('Ctrl Pts',(10.4681436286308,-1.08420482079362,0.7));
#11960=CARTESIAN_POINT('Ctrl Pts',(10.3770124662346,-1.0891584122264,0.7));
#11961=CARTESIAN_POINT('Ctrl Pts',(10.285877616441,-1.09404209584202,0.7));
#11962=CARTESIAN_POINT('Ctrl Pts',(10.1947388861048,-1.09885088260188,0.7));
#11963=CARTESIAN_POINT('Ctrl Pts',(10.4697107510168,-1.11303515260326,0.7));
#11964=CARTESIAN_POINT('Ctrl Pts',(10.3785648662465,-1.11799094453753,0.700000051218742));
#11965=CARTESIAN_POINT('Ctrl Pts',(10.2874149314686,-1.12287675076168,0.699999949550842));
#11966=CARTESIAN_POINT('Ctrl Pts',(10.196260416419,-1.12768774893097,0.7));
#11967=CARTESIAN_POINT('Ctrl Pts',(10.4724269697127,-1.16300539549315,0.676698381019543));
#11968=CARTESIAN_POINT('Ctrl Pts',(10.3812557252598,-1.16796482352885,0.676696026813929));
#11969=CARTESIAN_POINT('Ctrl Pts',(10.2900793016129,-1.17285439035486,0.676693724638983));
#11970=CARTESIAN_POINT('Ctrl Pts',(10.1988975981852,-1.17766904563614,0.67669140632491));
#11971=CARTESIAN_POINT('Ctrl Pts',(10.4734985149421,-1.18271860027509,0.627116141711795));
#11972=CARTESIAN_POINT('Ctrl Pts',(10.382317043787,-1.18767684023183,0.627110048826767));
#11973=CARTESIAN_POINT('Ctrl Pts',(10.2911301919381,-1.19256517083271,0.627104033151799));
#11974=CARTESIAN_POINT('Ctrl Pts',(10.1999375452555,-1.19737868557977,0.627098033786781));
#11975=CARTESIAN_POINT('Ctrl Pts',(10.4735630903435,-1.18390659316268,0.605494180667944));
#11976=CARTESIAN_POINT('Ctrl Pts',(10.3823809652617,-1.18886335120032,0.605486986548286));
#11977=CARTESIAN_POINT('Ctrl Pts',(10.2911933328565,-1.19375025772558,0.605479840815741));
#11978=CARTESIAN_POINT('Ctrl Pts',(10.1999999975038,-1.19856231440453,0.605472757505366));
#11979=CARTESIAN_POINT('',(10.4681436258201,-1.08420482094639,0.7));
#11980=CARTESIAN_POINT('Ctrl Pts',(10.4681436258201,-1.0842048209464,0.7));
#11981=CARTESIAN_POINT('Ctrl Pts',(10.3787660248044,-1.08906309452597,0.7));
#11982=CARTESIAN_POINT('Ctrl Pts',(10.289384876933,-1.09385412476048,0.7));
#11983=CARTESIAN_POINT('Ctrl Pts',(10.1999999999973,-1.09857320510493,0.7));
#11984=CARTESIAN_POINT('Origin',(10.4681436286308,-1.08420482099672,0.6));
#11985=CARTESIAN_POINT('Origin',(5.4,-8.11656130105013E-18,0.7));
#11986=CARTESIAN_POINT('',(10.4681436286308,1.08420482109828,0.7));
#11987=CARTESIAN_POINT('Ctrl Pts',(10.1999999980461,1.09857320520795,0.7));
#11988=CARTESIAN_POINT('Ctrl Pts',(10.2893848765692,1.09385412478074,0.7));
#11989=CARTESIAN_POINT('Ctrl Pts',(10.3787660260279,1.08906309446088,0.7));
#11990=CARTESIAN_POINT('Ctrl Pts',(10.4681436286308,1.08420482079361,0.7));
#11991=CARTESIAN_POINT('',(10.4681436286308,0.7,0.7));
#11992=CARTESIAN_POINT('Ctrl Pts',(7.3,1.35236351479305,-3.57463069561303E-11));
#11993=CARTESIAN_POINT('Ctrl Pts',(7.29625341766908,1.34178092325856,0.20193409200674));
#11994=CARTESIAN_POINT('Ctrl Pts',(7.29250676907475,1.33119833465113,0.403868182976914));
#11995=CARTESIAN_POINT('Ctrl Pts',(7.28876005303626,1.32061574904014,0.60580227285657));
#11996=CARTESIAN_POINT('Ctrl Pts',(8.20875307682014,1.32613868191819,-8.19770140467192E-5));
#11997=CARTESIAN_POINT('Ctrl Pts',(8.20321812688841,1.31555630757352,0.201851960063995));
#11998=CARTESIAN_POINT('Ctrl Pts',(8.19768309032092,1.3049739355521,0.403785895138154));
#11999=CARTESIAN_POINT('Ctrl Pts',(8.19214796413082,1.29439157094932,0.605719828284144));
#12000=CARTESIAN_POINT('Ctrl Pts',(9.11786336174626,1.28732002675385,-0.000205293251048056));
#12001=CARTESIAN_POINT('Ctrl Pts',(9.11054075262572,1.27673792860073,0.201728409716354));
#12002=CARTESIAN_POINT('Ctrl Pts',(9.10321803982063,1.26615583517412,0.403662109357089));
#12003=CARTESIAN_POINT('Ctrl Pts',(9.09589522044026,1.25557375159787,0.605595805709147));
#12004=CARTESIAN_POINT('Ctrl Pts',(10.0273290644402,1.2407389515511,-0.000342977407187712));
#12005=CARTESIAN_POINT('Ctrl Pts',(10.0182194939295,1.23015709330624,0.201590462897949));
#12006=CARTESIAN_POINT('Ctrl Pts',(10.0091098064748,1.21957524432641,0.403523898424684));
#12007=CARTESIAN_POINT('Ctrl Pts',(10.,1.20899340483035,0.605457329091028));
#12008=CARTESIAN_POINT('Ctrl Pts',(10.2,1.23178301601276,-2.39624899783797E-11));
#12009=CARTESIAN_POINT('Ctrl Pts',(10.1905551755807,1.22120572247504,0.201847146346486));
#12010=CARTESIAN_POINT('Ctrl Pts',(10.1811102319479,1.21062843858352,0.403694287656288));
#12011=CARTESIAN_POINT('Ctrl Pts',(10.1716651669865,1.2000511645658,0.605541423818621));
#12012=CARTESIAN_POINT('Ctrl Pts',(10.3017512542641,1.22646400658951,-1.55944220863836E-5));
#12013=CARTESIAN_POINT('Ctrl Pts',(10.2921066085356,1.2158867394917,0.201831522196997));
#12014=CARTESIAN_POINT('Ctrl Pts',(10.2824618422272,1.20530948226672,0.403678633585648));
#12015=CARTESIAN_POINT('Ctrl Pts',(10.2728169531999,1.19473223514819,0.605525739654127));
#12016=CARTESIAN_POINT('Ctrl Pts',(10.4035069533242,1.22105168617711,-3.13468015701665E-5));
#12017=CARTESIAN_POINT('Ctrl Pts',(10.3936624949945,1.21047444506608,0.201815739750419));
#12018=CARTESIAN_POINT('Ctrl Pts',(10.3838179147698,1.19989721405077,0.40366282090032));
#12019=CARTESIAN_POINT('Ctrl Pts',(10.3739732104878,1.18931999337006,0.605509896555428));
#12020=CARTESIAN_POINT('Ctrl Pts',(10.5052670937653,1.21555282972323,-4.72191118859062E-5));
#12021=CARTESIAN_POINT('Ctrl Pts',(10.495222831523,1.20497561405169,0.201799837128814));
#12022=CARTESIAN_POINT('Ctrl Pts',(10.4851784461213,1.19439840869429,0.403646887794301));
#12023=CARTESIAN_POINT('Ctrl Pts',(10.4751339353761,1.18382121389426,0.605493932788864));
#12024=CARTESIAN_POINT('',(10.4735630903435,1.18390659316268,0.605494180667944));
#12025=CARTESIAN_POINT('Ctrl Pts',(10.5052647440597,1.21555035534119,-4.0462425077159E-16));
#12026=CARTESIAN_POINT('Ctrl Pts',(10.4946974680575,1.20500226999407,0.201831382381129));
#12027=CARTESIAN_POINT('Ctrl Pts',(10.4841302498201,1.19445434834508,0.40366277587515));
#12028=CARTESIAN_POINT('Ctrl Pts',(10.4735630903435,1.18390659316268,0.605494180667945));
#12029=CARTESIAN_POINT('Ctrl Pts',(10.4735630903435,1.18390659316268,0.605494180667944));
#12030=CARTESIAN_POINT('Ctrl Pts',(10.3823809652617,1.18886335120032,0.605486986548286));
#12031=CARTESIAN_POINT('Ctrl Pts',(10.2911933328565,1.19375025772558,0.605479840815741));
#12032=CARTESIAN_POINT('Ctrl Pts',(10.1999999975038,1.19856231440453,0.605472757505366));
#12033=CARTESIAN_POINT('Origin',(7.1,1.42555555555556,0.));
#12034=CARTESIAN_POINT('',(7.0999999994629,-1.32593912634735,0.605276549957215));
#12035=CARTESIAN_POINT('Ctrl Pts',(7.0999999994629,-1.32593912634735,0.605276549957215));
#12036=CARTESIAN_POINT('Ctrl Pts',(7.0999999994629,-1.33126650931098,0.504490734647167));
#12037=CARTESIAN_POINT('Ctrl Pts',(7.1,-1.33659376385849,0.403703958452373));
#12038=CARTESIAN_POINT('Ctrl Pts',(7.1,-1.3472576786761,0.201945747207886));
#12039=CARTESIAN_POINT('Ctrl Pts',(7.1,-1.35259443928223,0.100972400854069));
#12040=CARTESIAN_POINT('Ctrl Pts',(7.1,-1.35793097395724,0.));
#12041=CARTESIAN_POINT('',(7.1,-1.22604182196417,0.7));
#12042=CARTESIAN_POINT('Ctrl Pts',(7.1,-1.22604182196307,0.7));
#12043=CARTESIAN_POINT('Ctrl Pts',(7.1,-1.23395163718705,0.7));
#12044=CARTESIAN_POINT('Ctrl Pts',(7.09999945440688,-1.24179783218049,0.699006056038995));
#12045=CARTESIAN_POINT('Ctrl Pts',(7.09999897931553,-1.2494401870438,0.697119011207626));
#12046=CARTESIAN_POINT('Ctrl Pts',(7.09999871186578,-1.25374240366384,0.696056710937424));
#12047=CARTESIAN_POINT('Ctrl Pts',(7.09999846845149,-1.25798007942473,0.69471034534287));
#12048=CARTESIAN_POINT('Ctrl Pts',(7.09999831430822,-1.26212651101681,0.6930909329195));
#12049=CARTESIAN_POINT('Ctrl Pts',(7.09999803835695,-1.26954956016987,0.690191818885951));
#12050=CARTESIAN_POINT('Ctrl Pts',(7.09999810102228,-1.27659977900265,0.686452252582521));
#12051=CARTESIAN_POINT('Ctrl Pts',(7.09999845706054,-1.28313109767173,0.681953977461377));
#12052=CARTESIAN_POINT('Ctrl Pts',(7.09999865314126,-1.2867280867584,0.679476645189077));
#12053=CARTESIAN_POINT('Ctrl Pts',(7.09999893113315,-1.29016742765117,0.67676830886676));
#12054=CARTESIAN_POINT('Ctrl Pts',(7.09999917787259,-1.2934208019838,0.673837071833988));
#12055=CARTESIAN_POINT('Ctrl Pts',(7.09999941835505,-1.29659167515528,0.670980166997299));
#12056=CARTESIAN_POINT('Ctrl Pts',(7.09999963169439,-1.29956664557352,0.667928795646746));
#12057=CARTESIAN_POINT('Ctrl Pts',(7.09999963110542,-1.30232317314677,0.664694459428825));
#12058=CARTESIAN_POINT('Ctrl Pts',(7.09999963001387,-1.30743194453681,0.658700148145236));
#12059=CARTESIAN_POINT('Ctrl Pts',(7.09999897381858,-1.31179333085743,0.652078782729069));
#12060=CARTESIAN_POINT('Ctrl Pts',(7.09999874753952,-1.31534789998199,0.64499600756552));
#12061=CARTESIAN_POINT('Ctrl Pts',(7.09999872438549,-1.31571162172319,0.644271261689237));
#12062=CARTESIAN_POINT('Ctrl Pts',(7.0999987046402,-1.31606685549941,0.643541664816448));
#12063=CARTESIAN_POINT('Ctrl Pts',(7.09999868869212,-1.31641350913238,0.642807383257706));
#12064=CARTESIAN_POINT('Ctrl Pts',(7.09999853283271,-1.31980133087414,0.635631300872562));
#12065=CARTESIAN_POINT('Ctrl Pts',(7.09999885939544,-1.32233451509485,0.628092322434426));
#12066=CARTESIAN_POINT('Ctrl Pts',(7.09999934101855,-1.32395982399511,0.620358959365968));
#12067=CARTESIAN_POINT('Ctrl Pts',(7.09999964997549,-1.32500244522074,0.615398075635307));
#12068=CARTESIAN_POINT('Ctrl Pts',(7.09999999934316,-1.32567060646853,0.610356529630438));
#12069=CARTESIAN_POINT('Ctrl Pts',(7.09999999981141,-1.32593912630714,0.60527654995744));
#12070=CARTESIAN_POINT('',(7.09999999995537,1.22604182196549,0.7));
#12071=CARTESIAN_POINT('',(7.1,0.712777777777778,0.7));
#12072=CARTESIAN_POINT('',(7.0999999994629,1.32593912634735,0.605276549957215));
#12073=CARTESIAN_POINT('Ctrl Pts',(7.09999999981142,1.32593912630714,0.60527654995744));
#12074=CARTESIAN_POINT('Ctrl Pts',(7.09999999908198,1.32552083177145,0.613190035045322));
#12075=CARTESIAN_POINT('Ctrl Pts',(7.09999922367565,1.32413525001942,0.621012727860624));
#12076=CARTESIAN_POINT('Ctrl Pts',(7.09999888117586,1.32186630199077,0.628584136488803));
#12077=CARTESIAN_POINT('Ctrl Pts',(7.09999868987568,1.32059900146923,0.632813078704371));
#12078=CARTESIAN_POINT('Ctrl Pts',(7.09999860640034,1.3190551184949,0.636963663611311));
#12079=CARTESIAN_POINT('Ctrl Pts',(7.09999865766138,1.31724253497577,0.641005923298765));
#12080=CARTESIAN_POINT('Ctrl Pts',(7.0999987494091,1.31399834762864,0.648240816253195));
#12081=CARTESIAN_POINT('Ctrl Pts',(7.09999933613984,1.30993159792479,0.655050690394837));
#12082=CARTESIAN_POINT('Ctrl Pts',(7.09999956222935,1.30510592187917,0.661272231165006));
#12083=CARTESIAN_POINT('Ctrl Pts',(7.09999960444598,1.30420484616769,0.662433950108221));
#12084=CARTESIAN_POINT('Ctrl Pts',(7.09999963060969,1.30327718139331,0.663575086117144));
#12085=CARTESIAN_POINT('Ctrl Pts',(7.09999963056866,1.30232317316131,0.664694459428815));
#12086=CARTESIAN_POINT('Ctrl Pts',(7.09999963048683,1.30042028596585,0.666927187690779));
#12087=CARTESIAN_POINT('Ctrl Pts',(7.09999952705857,1.29841262431024,0.669073382394206));
#12088=CARTESIAN_POINT('Ctrl Pts',(7.09999938633452,1.29630755303174,0.671129253595323));
#12089=CARTESIAN_POINT('Ctrl Pts',(7.09999900634735,1.29062337821964,0.676680576924663));
#12090=CARTESIAN_POINT('Ctrl Pts',(7.09999841760642,1.2842958957007,0.681513596217188));
#12091=CARTESIAN_POINT('Ctrl Pts',(7.0999982224057,1.2774887935492,0.68557385059291));
#12092=CARTESIAN_POINT('Ctrl Pts',(7.09999809840912,1.27316474526651,0.688153029745784));
#12093=CARTESIAN_POINT('Ctrl Pts',(7.09999810738417,1.26864620899217,0.690419707112974));
#12094=CARTESIAN_POINT('Ctrl Pts',(7.09999825155258,1.26396949224645,0.69235064530212));
#12095=CARTESIAN_POINT('Ctrl Pts',(7.09999847710269,1.25665281355793,0.695371579659609));
#12096=CARTESIAN_POINT('Ctrl Pts',(7.09999903441007,1.2490339950321,0.697538299034574));
#12097=CARTESIAN_POINT('Ctrl Pts',(7.09999948258254,1.24125996729125,0.698781081437474));
#12098=CARTESIAN_POINT('Ctrl Pts',(7.09999977198436,1.23623998534067,0.699583592753232));
#12099=CARTESIAN_POINT('Ctrl Pts',(7.1,1.23115469319345,0.7));
#12100=CARTESIAN_POINT('Ctrl Pts',(7.1,1.22604182196307,0.7));
#12101=CARTESIAN_POINT('Ctrl Pts',(7.1,1.35793097395724,0.));
#12102=CARTESIAN_POINT('Ctrl Pts',(7.1,1.35259441576718,0.100972845781549));
#12103=CARTESIAN_POINT('Ctrl Pts',(7.1,1.34725763161617,0.201946637598055));
#12104=CARTESIAN_POINT('Ctrl Pts',(7.1,1.33659371676552,0.403704849408333));
#12105=CARTESIAN_POINT('Ctrl Pts',(7.0999999994629,1.33126648576411,0.504491180117376));
#12106=CARTESIAN_POINT('Ctrl Pts',(7.0999999994629,1.32593912634735,0.605276549957215));
#12107=CARTESIAN_POINT('Ctrl Pts',(7.11011156210589,-1.35766432821499,-9.27062925672982E-5));
#12108=CARTESIAN_POINT('Ctrl Pts',(7.10674110347764,-1.34708925835705,0.201697046690488));
#12109=CARTESIAN_POINT('Ctrl Pts',(7.10337058314201,-1.33651419103807,0.403486798779133));
#12110=CARTESIAN_POINT('Ctrl Pts',(7.09999999999996,-1.32593912631822,0.605276549958221));
#12111=CARTESIAN_POINT('Ctrl Pts',(5.9694837631095,-1.38835096090528,2.80675674898241E-6));
#12112=CARTESIAN_POINT('Ctrl Pts',(5.96835662351021,-1.37777563343505,0.201792740207853));
#12113=CARTESIAN_POINT('Ctrl Pts',(5.96722945517891,-1.3672003004237,0.40358267322573));
#12114=CARTESIAN_POINT('Ctrl Pts',(5.96610224583462,-1.35662497356325,0.605372606931572));
#12115=CARTESIAN_POINT('Ctrl Pts',(4.8294200007394,-1.39866452387306,3.01102374082134E-5));
#12116=CARTESIAN_POINT('Ctrl Pts',(4.83053730380309,-1.38808904115766,0.201820093264151));
#12117=CARTESIAN_POINT('Ctrl Pts',(4.83165461298617,-1.3775135517806,0.403610075973038));
#12118=CARTESIAN_POINT('Ctrl Pts',(4.83277191472125,-1.36693806692183,0.605400059795761));
#12119=CARTESIAN_POINT('Ctrl Pts',(3.68991216363982,-1.37907703205181,-6.2684699445455E-5));
#12120=CARTESIAN_POINT('Ctrl Pts',(3.69327498756969,-1.36850179198701,0.201727122618256));
#12121=CARTESIAN_POINT('Ctrl Pts',(3.69663785098144,-1.3579265529724,0.403516929334346));
#12122=CARTESIAN_POINT('Ctrl Pts',(3.70000075457889,-1.34735131503281,0.605306735438421));
#12123=CARTESIAN_POINT('Ctrl Pts',(3.69999999992215,-1.34735368792773,0.6052614572053));
#12124=CARTESIAN_POINT('Ctrl Pts',(4.83355316856959,-1.366961322855,0.605214762857233));
#12125=CARTESIAN_POINT('Ctrl Pts',(5.96724522208681,-1.35660163688233,0.605228569880684));
#12126=CARTESIAN_POINT('Ctrl Pts',(7.09999999927392,-1.32593912632169,0.605276549957417));
#12127=CARTESIAN_POINT('Ctrl Pts',(7.1,-1.22604182196307,0.7));
#12128=CARTESIAN_POINT('Ctrl Pts',(5.96696284938742,-1.25674179781664,0.7));
#12129=CARTESIAN_POINT('Ctrl Pts',(4.83327074934872,-1.26710800714677,0.7));
#12130=CARTESIAN_POINT('Ctrl Pts',(3.7,-1.24747724070879,0.7));
#12131=CARTESIAN_POINT('Ctrl Pts',(7.10078315634008,-1.25494559805327,0.7));
#12132=CARTESIAN_POINT('Ctrl Pts',(5.96739926106349,-1.28566432005869,0.700000343763215));
#12133=CARTESIAN_POINT('Ctrl Pts',(4.83328164159484,-1.29603890521481,0.700000334703603));
#12134=CARTESIAN_POINT('Ctrl Pts',(3.69949916377151,-1.27639017438114,0.7));
#12135=CARTESIAN_POINT('Ctrl Pts',(7.10214055788579,-1.30504291366416,0.676629771601708));
#12136=CARTESIAN_POINT('Ctrl Pts',(5.96815960929481,-1.33579288254824,0.676614006760374));
#12137=CARTESIAN_POINT('Ctrl Pts',(4.83329467960724,-1.3461818279488,0.676609489640654));
#12138=CARTESIAN_POINT('Ctrl Pts',(3.69863109538965,-1.3265031696486,0.676624836591801));
#12139=CARTESIAN_POINT('Ctrl Pts',(7.10267376869946,-1.32472200604796,0.626932241521275));
#12140=CARTESIAN_POINT('Ctrl Pts',(5.9684558952243,-1.35546668061705,0.626891484245174));
#12141=CARTESIAN_POINT('Ctrl Pts',(4.83330292199863,-1.36585610284781,0.626879766983475));
#12142=CARTESIAN_POINT('Ctrl Pts',(3.69829020046733,-1.34618280086838,0.626919440930842));
#12143=CARTESIAN_POINT('Ctrl Pts',(7.10270476209941,-1.32586587253612,0.605276664588022));
#12144=CARTESIAN_POINT('Ctrl Pts',(5.96847377630401,-1.35660073810322,0.605228567467576));
#12145=CARTESIAN_POINT('Ctrl Pts',(4.8333022084086,-1.36698748587873,0.605214711607465));
#12146=CARTESIAN_POINT('Ctrl Pts',(3.69827043673666,-1.34732374755196,0.60526152849799));
#12147=CARTESIAN_POINT('Ctrl Pts',(7.1,-1.22604182196307,0.7));
#12148=CARTESIAN_POINT('Ctrl Pts',(5.96696284938742,-1.25674179781664,0.7));
#12149=CARTESIAN_POINT('Ctrl Pts',(4.83327074934872,-1.26710800714677,0.7));
#12150=CARTESIAN_POINT('Ctrl Pts',(3.7,-1.24747724070879,0.7));
#12151=CARTESIAN_POINT('Origin',(5.4,-8.11656130105013E-18,0.7));
#12152=CARTESIAN_POINT('Ctrl Pts',(3.7,1.24747724070879,0.7));
#12153=CARTESIAN_POINT('Ctrl Pts',(4.83327074934871,1.26710800714677,0.7));
#12154=CARTESIAN_POINT('Ctrl Pts',(5.96696284938742,1.25674179781664,0.7));
#12155=CARTESIAN_POINT('Ctrl Pts',(7.1,1.22604182196307,0.7));
#12156=CARTESIAN_POINT('Ctrl Pts',(3.7,1.24747724070879,0.7));
#12157=CARTESIAN_POINT('Ctrl Pts',(4.83327074934871,1.26710800714677,0.7));
#12158=CARTESIAN_POINT('Ctrl Pts',(5.96696284938742,1.25674179781664,0.7));
#12159=CARTESIAN_POINT('Ctrl Pts',(7.1,1.22604182196307,0.7));
#12160=CARTESIAN_POINT('Ctrl Pts',(3.69949916377151,1.27639017438114,0.7));
#12161=CARTESIAN_POINT('Ctrl Pts',(4.83328164159484,1.29603890521481,0.700000334703603));
#12162=CARTESIAN_POINT('Ctrl Pts',(5.96739926106349,1.28566432005869,0.700000343763215));
#12163=CARTESIAN_POINT('Ctrl Pts',(7.10078315634008,1.25494559805327,0.7));
#12164=CARTESIAN_POINT('Ctrl Pts',(3.69863109538965,1.3265031696486,0.676624836591801));
#12165=CARTESIAN_POINT('Ctrl Pts',(4.83329467960724,1.3461818279488,0.676609489640654));
#12166=CARTESIAN_POINT('Ctrl Pts',(5.9681596092948,1.33579288254824,0.676614006760374));
#12167=CARTESIAN_POINT('Ctrl Pts',(7.10214055788579,1.30504291366416,0.676629771601707));
#12168=CARTESIAN_POINT('Ctrl Pts',(3.69829020046733,1.34618280086838,0.626919440930842));
#12169=CARTESIAN_POINT('Ctrl Pts',(4.83330292199863,1.36585610284781,0.626879766983475));
#12170=CARTESIAN_POINT('Ctrl Pts',(5.9684558952243,1.35546668061705,0.626891484245174));
#12171=CARTESIAN_POINT('Ctrl Pts',(7.10267376869946,1.32472200604796,0.626932241521275));
#12172=CARTESIAN_POINT('Ctrl Pts',(3.69827043673666,1.34732374755196,0.60526152849799));
#12173=CARTESIAN_POINT('Ctrl Pts',(4.83330220840859,1.36698748587873,0.605214711607465));
#12174=CARTESIAN_POINT('Ctrl Pts',(5.96847377630401,1.35660073810322,0.605228567467576));
#12175=CARTESIAN_POINT('Ctrl Pts',(7.10270476209941,1.32586587253612,0.605276664588022));
#12176=CARTESIAN_POINT('Ctrl Pts',(7.09999999927392,1.32593912632169,0.605276549957417));
#12177=CARTESIAN_POINT('Ctrl Pts',(5.96724522208681,1.35660163688233,0.605228569880684));
#12178=CARTESIAN_POINT('Ctrl Pts',(4.83355316856959,1.366961322855,0.605214762857233));
#12179=CARTESIAN_POINT('Ctrl Pts',(3.69999999992215,1.34735368792773,0.6052614572053));
#12180=CARTESIAN_POINT('Ctrl Pts',(3.68991216360307,1.37907703216746,-6.26869063400631E-5));
#12181=CARTESIAN_POINT('Ctrl Pts',(3.6932749875452,1.36850179206412,0.201727121146993));
#12182=CARTESIAN_POINT('Ctrl Pts',(3.69663785096921,1.35792655301095,0.403516928598715));
#12183=CARTESIAN_POINT('Ctrl Pts',(3.70000075457892,1.34735131503281,0.605306735438421));
#12184=CARTESIAN_POINT('Ctrl Pts',(4.8294200007272,1.39866452398872,3.01080305115927E-5));
#12185=CARTESIAN_POINT('Ctrl Pts',(4.83053730379496,1.38808904123477,0.201820091792887));
#12186=CARTESIAN_POINT('Ctrl Pts',(4.83165461298211,1.37751355181915,0.403610075237406));
#12187=CARTESIAN_POINT('Ctrl Pts',(4.83277191472127,1.36693806692183,0.605400059795761));
#12188=CARTESIAN_POINT('Ctrl Pts',(5.96948376312183,1.38835096102094,2.80454985295556E-6));
#12189=CARTESIAN_POINT('Ctrl Pts',(5.96835662351844,1.37777563351215,0.201792738736588));
#12190=CARTESIAN_POINT('Ctrl Pts',(5.96722945518303,1.36720030046225,0.403582672490098));
#12191=CARTESIAN_POINT('Ctrl Pts',(5.96610224583462,1.35662497356325,0.605372606931572));
#12192=CARTESIAN_POINT('Ctrl Pts',(7.11011156214274,1.35766432833065,-9.27084994613511E-5));
#12193=CARTESIAN_POINT('Ctrl Pts',(7.10674110350221,1.34708925843416,0.201697045219225));
#12194=CARTESIAN_POINT('Ctrl Pts',(7.10337058315429,1.33651419107662,0.403486798043502));
#12195=CARTESIAN_POINT('Ctrl Pts',(7.09999999999996,1.32593912631822,0.605276549958221));
#12196=CARTESIAN_POINT('Origin',(3.5,1.44777777777778,0.));
#12197=CARTESIAN_POINT('',(3.5,-1.34358136363184,0.605270327458634));
#12198=CARTESIAN_POINT('Ctrl Pts',(3.5,-1.34358136363184,0.605270327458634));
#12199=CARTESIAN_POINT('Ctrl Pts',(3.5,-1.34890136370362,0.504489156176152));
#12200=CARTESIAN_POINT('Ctrl Pts',(3.5,-1.35422123464986,0.403706701640381));
#12201=CARTESIAN_POINT('Ctrl Pts',(3.5,-1.3648706701715,0.201950780690867));
#12202=CARTESIAN_POINT('Ctrl Pts',(3.5,-1.3702003690246,0.100974756199658));
#12203=CARTESIAN_POINT('Ctrl Pts',(3.5,-1.37552980833516,0.));
#12204=CARTESIAN_POINT('',(3.5,-1.24369946473884,0.7));
#12205=CARTESIAN_POINT('Ctrl Pts',(3.49999999991873,-1.24369946470729,0.7));
#12206=CARTESIAN_POINT('Ctrl Pts',(3.49999999896975,-1.25160831520001,0.699999999810925));
#12207=CARTESIAN_POINT('Ctrl Pts',(3.50000040534574,-1.25945374057332,0.69900619751828));
#12208=CARTESIAN_POINT('Ctrl Pts',(3.50000075715473,-1.26709539726361,0.697119355224275));
#12209=CARTESIAN_POINT('Ctrl Pts',(3.5000009551612,-1.27139630362835,0.696057395447694));
#12210=CARTESIAN_POINT('Ctrl Pts',(3.50000113454144,-1.27563271975905,0.694711510656402));
#12211=CARTESIAN_POINT('Ctrl Pts',(3.50000124621709,-1.27977793997275,0.693092697679401));
#12212=CARTESIAN_POINT('Ctrl Pts',(3.50000144618968,-1.28720060051191,0.690193961644836));
#12213=CARTESIAN_POINT('Ctrl Pts',(3.50000138985083,-1.29425038514255,0.686454755369034));
#12214=CARTESIAN_POINT('Ctrl Pts',(3.5000011147959,-1.30078112659466,0.681956784255818));
#12215=CARTESIAN_POINT('Ctrl Pts',(3.50000096334461,-1.30437709646577,0.679480102439082));
#12216=CARTESIAN_POINT('Ctrl Pts',(3.50000075087427,-1.30781543681835,0.676772489296601));
#12217=CARTESIAN_POINT('Ctrl Pts',(3.50000056308077,-1.31106783354026,0.67384203444854));
#12218=CARTESIAN_POINT('Ctrl Pts',(3.50000037990614,-1.31424023611357,0.670983655445047));
#12219=CARTESIAN_POINT('Ctrl Pts',(3.50000021841608,-1.31721646102264,0.667930553458483));
#12220=CARTESIAN_POINT('Ctrl Pts',(3.50000022028926,-1.3199739184757,0.664694242102541));
#12221=CARTESIAN_POINT('Ctrl Pts',(3.50000022375892,-1.32508151834405,0.658699667848218));
#12222=CARTESIAN_POINT('Ctrl Pts',(3.50000072745304,-1.32944146850927,0.652077914129702));
#12223=CARTESIAN_POINT('Ctrl Pts',(3.50000090782832,-1.33299465793893,0.64499486611401));
#12224=CARTESIAN_POINT('Ctrl Pts',(3.50000092626355,-1.33335781125732,0.644270944003422));
#12225=CARTESIAN_POINT('Ctrl Pts',(3.50000094214549,-1.33371249714824,0.643542183465449));
#12226=CARTESIAN_POINT('Ctrl Pts',(3.5000009551778,-1.33405862411533,0.642808750463418));
#12227=CARTESIAN_POINT('Ctrl Pts',(3.50000108270827,-1.3374457225345,0.635631587173848));
#12228=CARTESIAN_POINT('Ctrl Pts',(3.5000008470667,-1.33997810357527,0.628091493562486));
#12229=CARTESIAN_POINT('Ctrl Pts',(3.50000049017339,-1.34160279315579,0.620357239364781));
#12230=CARTESIAN_POINT('Ctrl Pts',(3.50000026118253,-1.3426452308862,0.615394766232079));
#12231=CARTESIAN_POINT('Ctrl Pts',(3.5,-1.34331313055125,0.610351689051435));
#12232=CARTESIAN_POINT('Ctrl Pts',(3.5,-1.34358136363184,0.605270327458634));
#12233=CARTESIAN_POINT('',(3.5,0.723888888888889,0.7));
#12234=CARTESIAN_POINT('Ctrl Pts',(3.5,1.37552980833516,0.));
#12235=CARTESIAN_POINT('Ctrl Pts',(3.5,1.37020035376703,0.10097504527886));
#12236=CARTESIAN_POINT('Ctrl Pts',(3.5,1.36487063968137,0.201951358354439));
#12237=CARTESIAN_POINT('Ctrl Pts',(3.5,1.35422120417274,0.403707279015233));
#12238=CARTESIAN_POINT('Ctrl Pts',(3.5,1.34890134846466,0.504489444860456));
#12239=CARTESIAN_POINT('Ctrl Pts',(3.5,1.34358136363184,0.605270327458635));
#12240=CARTESIAN_POINT('Ctrl Pts',(3.50000000097418,-1.37552980835478,3.46944695195361E-18));
#12241=CARTESIAN_POINT('Ctrl Pts',(3.50374047168104,-1.36494504174376,0.201972406882836));
#12242=CARTESIAN_POINT('Ctrl Pts',(3.50748098869546,-1.35436027657305,0.403944812985359));
#12243=CARTESIAN_POINT('Ctrl Pts',(3.51122155284351,-1.34377551287676,0.605917218294091));
#12244=CARTESIAN_POINT('Ctrl Pts',(2.69119625874569,-1.35924722858667,-7.54309614812119E-5));
#12245=CARTESIAN_POINT('Ctrl Pts',(2.69653217397324,-1.34866266892899,0.20189683354744));
#12246=CARTESIAN_POINT('Ctrl Pts',(2.70186816749714,-1.3380781117335,0.403869096002786));
#12247=CARTESIAN_POINT('Ctrl Pts',(2.7072042346663,-1.32749355863083,0.605841357314298));
#12248=CARTESIAN_POINT('Ctrl Pts',(1.88267190563219,-1.32763345268679,-0.000212792412547521));
#12249=CARTESIAN_POINT('Ctrl Pts',(1.88960380459144,-1.31704931403188,0.201759213581099));
#12250=CARTESIAN_POINT('Ctrl Pts',(1.89653581411498,-1.30646518166523,0.403731216009517));
#12251=CARTESIAN_POINT('Ctrl Pts',(1.90346792975642,-1.29588105699583,0.605703215867581));
#12252=CARTESIAN_POINT('Ctrl Pts',(1.07441451989529,-1.27728918272486,-0.000429194541766893));
#12253=CARTESIAN_POINT('Ctrl Pts',(1.08294287068452,-1.26670581246828,0.201542410257184));
#12254=CARTESIAN_POINT('Ctrl Pts',(1.09147136321593,-1.25612245578053,0.403514009799157));
#12255=CARTESIAN_POINT('Ctrl Pts',(1.09999999999989,-1.24553911298205,0.605485603995245));
#12256=CARTESIAN_POINT('Ctrl Pts',(1.09999999916631,-1.24553911263844,0.605485603997431));
#12257=CARTESIAN_POINT('Ctrl Pts',(1.89930203168262,-1.29563783986497,0.605377360150118));
#12258=CARTESIAN_POINT('Ctrl Pts',(2.69958486793449,-1.32722445934619,0.605308375488923));
#12259=CARTESIAN_POINT('Ctrl Pts',(3.5,-1.34358136363184,0.605270327458634));
#12260=CARTESIAN_POINT('Ctrl Pts',(3.50204003610941,-1.24374118183538,0.7));
#12261=CARTESIAN_POINT('Ctrl Pts',(2.70080437300401,-1.2273695200909,0.7));
#12262=CARTESIAN_POINT('Ctrl Pts',(1.89984199608574,-1.1957170361627,0.7));
#12263=CARTESIAN_POINT('Ctrl Pts',(1.1,-1.14549341399196,0.7));
#12264=CARTESIAN_POINT('Ctrl Pts',(3.50144932661635,-1.27265074030048,0.7));
#12265=CARTESIAN_POINT('Ctrl Pts',(2.6998452019678,-1.25626413437997,0.699999727319846));
#12266=CARTESIAN_POINT('Ctrl Pts',(1.89847848223078,-1.22458382597074,0.70000077422621));
#12267=CARTESIAN_POINT('Ctrl Pts',(1.09819048660397,-1.17431102498992,0.7));
#12268=CARTESIAN_POINT('Ctrl Pts',(3.50042536655637,-1.322763754511,0.676632802377821));
#12269=CARTESIAN_POINT('Ctrl Pts',(2.69818680938114,-1.3063522351595,0.67664530655333));
#12270=CARTESIAN_POINT('Ctrl Pts',(1.89610976425884,-1.27462253270773,0.67666760713801));
#12271=CARTESIAN_POINT('Ctrl Pts',(1.09505363188407,-1.22426736091617,0.676703190608825));
#12272=CARTESIAN_POINT('Ctrl Pts',(3.50002334924346,-1.34243864233338,0.626926882269943));
#12273=CARTESIAN_POINT('Ctrl Pts',(2.6975332861013,-1.32603127467068,0.626959208652505));
#12274=CARTESIAN_POINT('Ctrl Pts',(1.89518106151152,-1.29430885982199,0.62701751976321));
#12275=CARTESIAN_POINT('Ctrl Pts',(1.09381704710221,-1.24396073223232,0.627109609335854));
#12276=CARTESIAN_POINT('Ctrl Pts',(3.5,-1.34358136363184,0.605270327458634));
#12277=CARTESIAN_POINT('Ctrl Pts',(2.69749615303,-1.32718177535833,0.605308474776761));
#12278=CARTESIAN_POINT('Ctrl Pts',(1.89512529323683,-1.29547288309274,0.605377720397184));
#12279=CARTESIAN_POINT('Ctrl Pts',(1.09374258853658,-1.24514653057163,0.605486452199395));
#12280=CARTESIAN_POINT('Ctrl Pts',(3.49999999991875,-1.24369946470729,0.7));
#12281=CARTESIAN_POINT('Ctrl Pts',(3.26917843083003,-1.23897560807887,0.7));
#12282=CARTESIAN_POINT('Ctrl Pts',(3.03837960179139,-1.23298334389983,0.7));
#12283=CARTESIAN_POINT('Ctrl Pts',(2.80762376541487,-1.22564400623233,0.7));
#12284=CARTESIAN_POINT('Ctrl Pts',(2.57739190516312,-1.2178709162388,0.7));
#12285=CARTESIAN_POINT('Ctrl Pts',(2.08463535466707,-1.20026407570248,0.7));
#12286=CARTESIAN_POINT('Ctrl Pts',(1.59210562457525,-1.17639367564078,0.7));
#12287=CARTESIAN_POINT('Ctrl Pts',(1.1,-1.14549341399196,0.7));
#12288=CARTESIAN_POINT('Origin',(5.4,-8.11656130105013E-18,0.7));
#12289=CARTESIAN_POINT('Ctrl Pts',(1.0744145198953,1.27728918272486,-0.000429194541767127));
#12290=CARTESIAN_POINT('Ctrl Pts',(1.08294287068452,1.26670581246828,0.201542410257184));
#12291=CARTESIAN_POINT('Ctrl Pts',(1.09147136321593,1.25612245578053,0.403514009799157));
#12292=CARTESIAN_POINT('Ctrl Pts',(1.0999999999999,1.24553911298205,0.605485603995245));
#12293=CARTESIAN_POINT('Ctrl Pts',(1.88267190563235,1.3276334526868,-0.000212792412547728));
#12294=CARTESIAN_POINT('Ctrl Pts',(1.8896038045916,1.31704931403189,0.201759213581098));
#12295=CARTESIAN_POINT('Ctrl Pts',(1.89653581411514,1.30646518166524,0.403731216009517));
#12296=CARTESIAN_POINT('Ctrl Pts',(1.90346792975658,1.29588105699584,0.605703215867581));
#12297=CARTESIAN_POINT('Ctrl Pts',(2.69119625874601,1.35924722858668,-7.54309614812134E-5));
#12298=CARTESIAN_POINT('Ctrl Pts',(2.69653217397356,1.348662668929,0.201896833547441));
#12299=CARTESIAN_POINT('Ctrl Pts',(2.70186816749745,1.33807811173351,0.403869096002786));
#12300=CARTESIAN_POINT('Ctrl Pts',(2.70720423466661,1.32749355863085,0.605841357314298));
#12301=CARTESIAN_POINT('Ctrl Pts',(3.50000000097466,1.37552980835479,-3.81639164714898E-17));
#12302=CARTESIAN_POINT('Ctrl Pts',(3.50374047168151,1.36494504174377,0.201972406882836));
#12303=CARTESIAN_POINT('Ctrl Pts',(3.50748098869594,1.35436027657306,0.403944812985359));
#12304=CARTESIAN_POINT('Ctrl Pts',(3.51122155284398,1.34377551287677,0.605917218294091));
#12305=CARTESIAN_POINT('Origin',(0.9,1.34328341716202,0.));
#12306=CARTESIAN_POINT('',(0.9,-1.23261418131727,0.605513513251856));
#12307=CARTESIAN_POINT('Ctrl Pts',(0.9,-1.23261418131727,0.605513513251856));
#12308=CARTESIAN_POINT('Ctrl Pts',(0.9,-1.23820195798151,0.504544236118289));
#12309=CARTESIAN_POINT('Ctrl Pts',(0.9,-1.24378834611607,0.403573587101897));
#12310=CARTESIAN_POINT('Ctrl Pts',(0.9,-1.25495246062481,0.201736610752668));
#12311=CARTESIAN_POINT('Ctrl Pts',(0.9,-1.26053033259331,0.100867703930409));
#12312=CARTESIAN_POINT('Ctrl Pts',(0.9,-1.266106713614,0.));
#12313=CARTESIAN_POINT('',(0.9,-1.13254484134404,0.7));
#12314=CARTESIAN_POINT('Ctrl Pts',(0.899999999937205,-1.13254484130906,
0.7));
#12315=CARTESIAN_POINT('Ctrl Pts',(0.899999996287105,-1.14047016437301,
0.699999998205918));
#12316=CARTESIAN_POINT('Ctrl Pts',(0.900001280561548,-1.14833327216777,
0.699006663725481));
#12317=CARTESIAN_POINT('Ctrl Pts',(0.900002371513522,-1.15599299513142,
0.697119896446058));
#12318=CARTESIAN_POINT('Ctrl Pts',(0.900002982478546,-1.16028266409831,
0.696063251566776));
#12319=CARTESIAN_POINT('Ctrl Pts',(0.900003528700818,-1.16450859688491,
0.694725368779139));
#12320=CARTESIAN_POINT('Ctrl Pts',(0.900003857331964,-1.16864431737637,
0.693116947675672));
#12321=CARTESIAN_POINT('Ctrl Pts',(0.900004447924614,-1.17607674172948,
0.690226407030055));
#12322=CARTESIAN_POINT('Ctrl Pts',(0.900004211500339,-1.18313828052408,
0.686496282267003));
#12323=CARTESIAN_POINT('Ctrl Pts',(0.900003280035406,-1.18968205680082,
0.682006679400108));
#12324=CARTESIAN_POINT('Ctrl Pts',(0.900002768383153,-1.19327654302499,
0.679540547464272));
#12325=CARTESIAN_POINT('Ctrl Pts',(0.900002064672634,-1.19671453445753,
0.676844382327844));
#12326=CARTESIAN_POINT('Ctrl Pts',(0.900001450170085,-1.19996775918788,
0.673925988054463));
#12327=CARTESIAN_POINT('Ctrl Pts',(0.900000850201302,-1.20314404102283,
0.67107661751105));
#12328=CARTESIAN_POINT('Ctrl Pts',(0.900000329673364,-1.20612495630093,
0.668032594545539));
#12329=CARTESIAN_POINT('Ctrl Pts',(0.900000346081477,-1.20888784276431,
0.664805176146368));
#12330=CARTESIAN_POINT('Ctrl Pts',(0.900000376514472,-1.21401231436848,
0.658819112599938));
#12331=CARTESIAN_POINT('Ctrl Pts',(0.900002057232535,-1.21838968018573,
0.652203523053766));
#12332=CARTESIAN_POINT('Ctrl Pts',(0.900002698394847,-1.22195969054856,
0.645123732731769));
#12333=CARTESIAN_POINT('Ctrl Pts',(0.900002763240662,-1.22232075393107,
0.644407697543824));
#12334=CARTESIAN_POINT('Ctrl Pts',(0.90000282009371,-1.22267351953901,0.643686895083047));
#12335=CARTESIAN_POINT('Ctrl Pts',(0.900002868017411,-1.22301789747605,
0.642961485862499));
#12336=CARTESIAN_POINT('Ctrl Pts',(0.900003341628975,-1.22642125256928,
0.635792544708285));
#12337=CARTESIAN_POINT('Ctrl Pts',(0.900002645022176,-1.22896979279554,
0.628258742918086));
#12338=CARTESIAN_POINT('Ctrl Pts',(0.900001532827652,-1.23061007098772,
0.6205286650049));
#12339=CARTESIAN_POINT('Ctrl Pts',(0.900000822323555,-1.23165793118585,
0.61559045329652));
#12340=CARTESIAN_POINT('Ctrl Pts',(0.900000000000001,-1.23233426661673,
0.610571479357261));
#12341=CARTESIAN_POINT('Ctrl Pts',(0.900000000000001,-1.23261418131727,
0.605513513251856));
#12342=CARTESIAN_POINT('',(0.9,1.13254484134404,0.7));
#12343=CARTESIAN_POINT('',(0.9,0.671641708581009,0.7));
#12344=CARTESIAN_POINT('',(0.9,1.23261418131727,0.605513513251856));
#12345=CARTESIAN_POINT('Ctrl Pts',(0.9,1.23261418131727,0.605513513251856));
#12346=CARTESIAN_POINT('Ctrl Pts',(0.9,1.23217633603244,0.613425232807268));
#12347=CARTESIAN_POINT('Ctrl Pts',(0.900001832787994,1.23077105609892,0.621244170085157));
#12348=CARTESIAN_POINT('Ctrl Pts',(0.900002580745575,1.22848219166492,0.628809599741497));
#12349=CARTESIAN_POINT('Ctrl Pts',(0.900002993068559,1.22722042035689,0.632980157827643));
#12350=CARTESIAN_POINT('Ctrl Pts',(0.90000314174678,1.22568915198244,0.637073706995481));
#12351=CARTESIAN_POINT('Ctrl Pts',(0.900002971484041,1.2238959908032,0.641061424759933));
#12352=CARTESIAN_POINT('Ctrl Pts',(0.900002662567364,1.22064256379503,0.648296551655426));
#12353=CARTESIAN_POINT('Ctrl Pts',(0.900001146653719,1.21656554418039,0.655104870690721));
#12354=CARTESIAN_POINT('Ctrl Pts',(0.900000540233788,1.21172928299109,0.66132323772617));
#12355=CARTESIAN_POINT('Ctrl Pts',(0.900000424918953,1.21080963534652,0.66250570210793));
#12356=CARTESIAN_POINT('Ctrl Pts',(0.900000351402035,1.20986240082127,0.663666762843393));
#12357=CARTESIAN_POINT('Ctrl Pts',(0.900000346234225,1.20888784277449,0.664805176146358));
#12358=CARTESIAN_POINT('Ctrl Pts',(0.900000336405833,1.20703438079614,0.666970266034709));
#12359=CARTESIAN_POINT('Ctrl Pts',(0.900000571869483,1.20508211779724,0.669053482241208));
#12360=CARTESIAN_POINT('Ctrl Pts',(0.900000903580486,1.20303784749416,0.671051418948595));
#12361=CARTESIAN_POINT('Ctrl Pts',(0.900001825932764,1.19735357006848,0.676606861644505));
#12362=CARTESIAN_POINT('Ctrl Pts',(0.900003332967427,1.19102482074992,0.681443262092019));
#12363=CARTESIAN_POINT('Ctrl Pts',(0.900003895332687,1.18421635668109,0.685507797106414));
#12364=CARTESIAN_POINT('Ctrl Pts',(0.900004254598985,1.17986677848026,0.688104419886002));
#12365=CARTESIAN_POINT('Ctrl Pts',(0.9000042929279,1.17532044218795,0.69038534615497));
#12366=CARTESIAN_POINT('Ctrl Pts',(0.900003997675654,1.17061445353731,0.692327416690341));
#12367=CARTESIAN_POINT('Ctrl Pts',(0.900003537640084,1.16328200409216,0.695353376818313));
#12368=CARTESIAN_POINT('Ctrl Pts',(0.900002259964378,1.15564663185935,0.697524398440697));
#12369=CARTESIAN_POINT('Ctrl Pts',(0.900001215101098,1.14785635641255,0.698771715080855));
#12370=CARTESIAN_POINT('Ctrl Pts',(0.900000537649455,1.14280542295857,0.699580430175527));
#12371=CARTESIAN_POINT('Ctrl Pts',(0.899999997568109,1.13768876957788,0.699999998835552));
#12372=CARTESIAN_POINT('Ctrl Pts',(0.899999999937205,1.13254484130906,0.7));
#12373=CARTESIAN_POINT('Ctrl Pts',(0.9,1.266106713614,0.));
#12374=CARTESIAN_POINT('Ctrl Pts',(0.9,1.26053025554556,0.100869097599589));
#12375=CARTESIAN_POINT('Ctrl Pts',(0.9,1.25495230648558,0.201739398169819));
#12376=CARTESIAN_POINT('Ctrl Pts',(0.9,1.24378819189631,0.403576374532447));
#12377=CARTESIAN_POINT('Ctrl Pts',(0.9,1.23820188085298,0.504545629805417));
#12378=CARTESIAN_POINT('Ctrl Pts',(0.9,1.23261418131727,0.605513513251856));
#12379=CARTESIAN_POINT('Ctrl Pts',(0.900000000000002,-1.266106713614,-8.15320033709099E-17));
#12380=CARTESIAN_POINT('Ctrl Pts',(0.908871090277923,-1.25552568177643,
0.201930159665972));
#12381=CARTESIAN_POINT('Ctrl Pts',(0.917742329685194,-1.24494466498547,
0.403860313587921));
#12382=CARTESIAN_POINT('Ctrl Pts',(0.926613720860141,-1.23436366359623,
0.605790461668883));
#12383=CARTESIAN_POINT('Ctrl Pts',(0.697441255022372,-1.25280938151844,
-5.71013218131409E-5));
#12384=CARTESIAN_POINT('Ctrl Pts',(0.706712389899261,-1.24222855501813,
0.201872952723963));
#12385=CARTESIAN_POINT('Ctrl Pts',(0.71598368260269,-1.23164774534186,0.403803000441224));
#12386=CARTESIAN_POINT('Ctrl Pts',(0.725255135891715,-1.22106695288555,
0.605733041729342));
#12387=CARTESIAN_POINT('Ctrl Pts',(0.494899146035781,-1.23832021354117,
-0.000119230777047918));
#12388=CARTESIAN_POINT('Ctrl Pts',(0.504570354086872,-1.2277396148863,0.201810708652083));
#12389=CARTESIAN_POINT('Ctrl Pts',(0.514241728780064,-1.21715903502506,
0.403740641123913));
#12390=CARTESIAN_POINT('Ctrl Pts',(0.523913273026478,-1.20657847439907,
0.605670566527588));
#12391=CARTESIAN_POINT('Ctrl Pts',(0.292373353339556,-1.22258574808743,
-0.000186633859775947));
#12392=CARTESIAN_POINT('Ctrl Pts',(0.302444661323169,-1.21200540195431,
0.201743181663441));
#12393=CARTESIAN_POINT('Ctrl Pts',(0.312516144861689,-1.20142507679253,
0.403672989556125));
#12394=CARTESIAN_POINT('Ctrl Pts',(0.322587807049886,-1.190844773096,0.605602789690272));
#12395=CARTESIAN_POINT('',(0.32407846024449,-1.19096124572524,0.605603291426262));
#12396=CARTESIAN_POINT('Ctrl Pts',(0.292382661757373,-1.22257596919059,
-1.26634813746307E-16));
#12397=CARTESIAN_POINT('Ctrl Pts',(0.302948004341657,-1.21203750712027,
0.201867748891544));
#12398=CARTESIAN_POINT('Ctrl Pts',(0.313513270922098,-1.20149926476964,
0.403735512620674));
#12399=CARTESIAN_POINT('Ctrl Pts',(0.324078460244491,-1.19096124572524,
0.605603291426262));
#12400=CARTESIAN_POINT('Ctrl Pts',(0.324078460244487,-1.19096124572524,
0.605603291426262));
#12401=CARTESIAN_POINT('Ctrl Pts',(0.515976798438381,-1.20595780001216,
0.605571001180369));
#12402=CARTESIAN_POINT('Ctrl Pts',(0.707956283694857,-1.21982772882273,
0.605541108414459));
#12403=CARTESIAN_POINT('Ctrl Pts',(0.900000000000001,-1.23261418131727,
0.605513513251856));
#12404=CARTESIAN_POINT('Ctrl Pts',(0.906632491847682,-1.13298681949577,
0.7));
#12405=CARTESIAN_POINT('Ctrl Pts',(0.714963137593258,-1.12022681655782,
0.7));
#12406=CARTESIAN_POINT('Ctrl Pts',(0.52336552158394,-1.10638609587519,0.7));
#12407=CARTESIAN_POINT('Ctrl Pts',(0.331856371369197,-1.09142177001972,
0.7));
#12408=CARTESIAN_POINT('Ctrl Pts',(0.904714827274509,-1.16179226195561,
0.7));
#12409=CARTESIAN_POINT('Ctrl Pts',(0.712937153454425,-1.14901967286075,
0.69999980360337));
#12410=CARTESIAN_POINT('Ctrl Pts',(0.521230340369869,-1.13516557394852,
0.700000229443053));
#12411=CARTESIAN_POINT('Ctrl Pts',(0.329608751265076,-1.12018616744754,
0.7));
#12412=CARTESIAN_POINT('Ctrl Pts',(0.901389714107723,-1.21173913866089,
0.676722045797292));
#12413=CARTESIAN_POINT('Ctrl Pts',(0.709425477581998,-1.19894546296063,
0.676731074746188));
#12414=CARTESIAN_POINT('Ctrl Pts',(0.517526696841433,-1.18506766126723,
0.67674067107047));
#12415=CARTESIAN_POINT('Ctrl Pts',(0.325711429829026,-1.17006296935233,
0.676751229163451));
#12416=CARTESIAN_POINT('Ctrl Pts',(0.900079298017777,-1.23142303740181,
0.627132481749528));
#12417=CARTESIAN_POINT('Ctrl Pts',(0.708040181852795,-1.21863106773591,
0.627155851652593));
#12418=CARTESIAN_POINT('Ctrl Pts',(0.516066269599777,-1.20475540724405,
0.627181012790208));
#12419=CARTESIAN_POINT('Ctrl Pts',(0.324172915772929,-1.18975243096407,
0.627208352638976));
#12420=CARTESIAN_POINT('Ctrl Pts',(0.900000000000001,-1.23261418131727,
0.605513513251856));
#12421=CARTESIAN_POINT('Ctrl Pts',(0.707956283694857,-1.21982772882273,
0.605541108414459));
#12422=CARTESIAN_POINT('Ctrl Pts',(0.515976798438381,-1.20595780001216,
0.605571001180369));
#12423=CARTESIAN_POINT('Ctrl Pts',(0.324078460244487,-1.19096124572524,
0.605603291426262));
#12424=CARTESIAN_POINT('',(0.3318563713692,-1.09142177001972,0.7));
#12425=CARTESIAN_POINT('Origin',(0.3318563713692,-1.09142177001972,0.6));
#12426=CARTESIAN_POINT('Ctrl Pts',(0.899999999937167,-1.13254484130906,
0.7));
#12427=CARTESIAN_POINT('Ctrl Pts',(0.710543123935439,-1.11990737114256,
0.7));
#12428=CARTESIAN_POINT('Ctrl Pts',(0.521156529292483,-1.10621348751457,
0.7));
#12429=CARTESIAN_POINT('Ctrl Pts',(0.331856371369197,-1.09142177001972,
0.7));
#12430=CARTESIAN_POINT('Origin',(5.4,-8.11656130105013E-18,0.7));
#12431=CARTESIAN_POINT('',(0.3318563713692,1.09142177001972,0.7));
#12432=CARTESIAN_POINT('',(0.3318563713692,-0.7,0.7));
#12433=CARTESIAN_POINT('Ctrl Pts',(0.3318563713692,1.09142177001972,0.7));
#12434=CARTESIAN_POINT('Ctrl Pts',(0.521156529292483,1.10621348751457,0.7));
#12435=CARTESIAN_POINT('Ctrl Pts',(0.710543123935438,1.11990737114256,0.7));
#12436=CARTESIAN_POINT('Ctrl Pts',(0.899999999937165,1.13254484130906,0.7));
#12437=CARTESIAN_POINT('Ctrl Pts',(0.292373353339556,1.22258574808743,-0.000186633859776018));
#12438=CARTESIAN_POINT('Ctrl Pts',(0.30244466132317,1.21200540195431,0.20174318166344));
#12439=CARTESIAN_POINT('Ctrl Pts',(0.31251614486169,1.20142507679253,0.403672989556124));
#12440=CARTESIAN_POINT('Ctrl Pts',(0.322587807049886,1.190844773096,0.605602789690271));
#12441=CARTESIAN_POINT('Ctrl Pts',(0.494899146035781,1.23832021354117,-0.000119230777047989));
#12442=CARTESIAN_POINT('Ctrl Pts',(0.504570354086872,1.2277396148863,0.201810708652083));
#12443=CARTESIAN_POINT('Ctrl Pts',(0.514241728780064,1.21715903502506,0.403740641123914));
#12444=CARTESIAN_POINT('Ctrl Pts',(0.523913273026478,1.20657847439907,0.605670566527587));
#12445=CARTESIAN_POINT('Ctrl Pts',(0.697441255022371,1.25280938151844,-5.71013218130602E-5));
#12446=CARTESIAN_POINT('Ctrl Pts',(0.70671238989926,1.24222855501813,0.201872952723963));
#12447=CARTESIAN_POINT('Ctrl Pts',(0.715983682602689,1.23164774534186,0.403803000441224));
#12448=CARTESIAN_POINT('Ctrl Pts',(0.725255135891714,1.22106695288555,0.605733041729342));
#12449=CARTESIAN_POINT('Ctrl Pts',(0.9,1.266106713614,1.73472347597681E-18));
#12450=CARTESIAN_POINT('Ctrl Pts',(0.908871090277921,1.25552568177643,0.201930159665973));
#12451=CARTESIAN_POINT('Ctrl Pts',(0.917742329685192,1.24494466498547,0.403860313587921));
#12452=CARTESIAN_POINT('Ctrl Pts',(0.92661372086014,1.23436366359623,0.605790461668883));
#12453=CARTESIAN_POINT('',(0.32407846024449,1.19096124572524,0.605603291426262));
#12454=CARTESIAN_POINT('Ctrl Pts',(0.9,1.23261418131727,0.605513513251856));
#12455=CARTESIAN_POINT('Ctrl Pts',(0.707956283694857,1.21982772882273,0.605541108414459));
#12456=CARTESIAN_POINT('Ctrl Pts',(0.515976798438382,1.20595780001216,0.60557100118037));
#12457=CARTESIAN_POINT('Ctrl Pts',(0.32407846024449,1.19096124572524,0.605603291426262));
#12458=CARTESIAN_POINT('Ctrl Pts',(0.324078460244491,1.19096124572524,0.605603291426262));
#12459=CARTESIAN_POINT('Ctrl Pts',(0.313513270922098,1.20149926476964,0.403735512620674));
#12460=CARTESIAN_POINT('Ctrl Pts',(0.302948004341658,1.21203750712026,0.201867748891544));
#12461=CARTESIAN_POINT('Ctrl Pts',(0.292382661757373,1.22257596919059,3.4477629085039E-17));
#12462=CARTESIAN_POINT('Ctrl Pts',(0.3318563713692,1.09142177001972,0.7));
#12463=CARTESIAN_POINT('Ctrl Pts',(0.523365521583941,1.10638609587519,0.7));
#12464=CARTESIAN_POINT('Ctrl Pts',(0.714963137593258,1.12022681655782,0.7));
#12465=CARTESIAN_POINT('Ctrl Pts',(0.906632491847681,1.13298681949577,0.7));
#12466=CARTESIAN_POINT('Ctrl Pts',(0.329608751265078,1.12018616744754,0.7));
#12467=CARTESIAN_POINT('Ctrl Pts',(0.52123034036987,1.13516557394852,0.700000229443053));
#12468=CARTESIAN_POINT('Ctrl Pts',(0.712937153454426,1.14901967286075,0.699999803603371));
#12469=CARTESIAN_POINT('Ctrl Pts',(0.904714827274509,1.16179226195561,0.700000000000001));
#12470=CARTESIAN_POINT('Ctrl Pts',(0.325711429829028,1.17006296935233,0.676751229163452));
#12471=CARTESIAN_POINT('Ctrl Pts',(0.517526696841433,1.18506766126723,0.67674067107047));
#12472=CARTESIAN_POINT('Ctrl Pts',(0.709425477581997,1.19894546296063,0.676731074746189));
#12473=CARTESIAN_POINT('Ctrl Pts',(0.901389714107722,1.21173913866089,0.676722045797292));
#12474=CARTESIAN_POINT('Ctrl Pts',(0.324172915772932,1.18975243096407,0.627208352638976));
#12475=CARTESIAN_POINT('Ctrl Pts',(0.516066269599778,1.20475540724405,0.627181012790208));
#12476=CARTESIAN_POINT('Ctrl Pts',(0.708040181852794,1.21863106773591,0.627155851652593));
#12477=CARTESIAN_POINT('Ctrl Pts',(0.900079298017776,1.23142303740181,0.627132481749528));
#12478=CARTESIAN_POINT('Ctrl Pts',(0.32407846024449,1.19096124572524,0.605603291426262));
#12479=CARTESIAN_POINT('Ctrl Pts',(0.515976798438382,1.20595780001216,0.60557100118037));
#12480=CARTESIAN_POINT('Ctrl Pts',(0.707956283694857,1.21982772882273,0.605541108414459));
#12481=CARTESIAN_POINT('Ctrl Pts',(0.9,1.23261418131727,0.605513513251856));
#12482=CARTESIAN_POINT('Origin',(0.331856371369202,1.09142177001972,0.6));
#12483=CARTESIAN_POINT('Origin',(0.331856371369202,1.09142177001972,0.6));
#12484=CARTESIAN_POINT('Origin',(0.331856371369201,1.09142177001972,0.6));
#12485=CARTESIAN_POINT('Origin',(0.331856371369202,1.09142177001972,0.6));
#12486=CARTESIAN_POINT('Origin',(10.4681436286308,1.08420482079361,0.6));
#12487=CARTESIAN_POINT('Origin',(10.4681436276939,1.08420482084454,0.6));
#12488=CARTESIAN_POINT('',(10.5680065821063,1.08420482079361,0.605233595624295));
#12489=CARTESIAN_POINT('Origin',(10.4681436286308,1.08420482079361,0.6));
#12490=CARTESIAN_POINT('Origin',(10.4681436286308,1.08420482079361,0.6));
#12491=CARTESIAN_POINT('Origin',(0.3318563713692,-1.09142177001972,0.6));
#12492=CARTESIAN_POINT('Origin',(0.331856371369201,-1.09142177001972,0.6));
#12493=CARTESIAN_POINT('Origin',(0.3318563713692,-1.09142177001972,0.6));
#12494=CARTESIAN_POINT('Origin',(0.3318563713692,-0.7,0.6));
#12495=CARTESIAN_POINT('Ctrl Pts',(0.2922895713475,-1.22266882276207,-0.00177864096060679));
#12496=CARTESIAN_POINT('Ctrl Pts',(0.302885944515497,-1.21209940820877,
0.200681988163859));
#12497=CARTESIAN_POINT('Ctrl Pts',(0.313482241236256,-1.20153021465708,
0.403142632212487));
#12498=CARTESIAN_POINT('Ctrl Pts',(0.324078460244491,-1.19096124572524,
0.605603291426262));
#12499=CARTESIAN_POINT('Ctrl Pts',(0.264022491930188,-1.22039553779506,
-0.000415890128406236));
#12500=CARTESIAN_POINT('Ctrl Pts',(0.274621881512248,-1.20982222712748,
0.202044379074236));
#12501=CARTESIAN_POINT('Ctrl Pts',(0.285221154833576,-1.19924944554801,
0.404504681968985));
#12502=CARTESIAN_POINT('Ctrl Pts',(0.29582042516239,-1.18867654001483,0.606964977361795));
#12503=CARTESIAN_POINT('Ctrl Pts',(0.216712469170969,-1.1940874043406,0.000690255297866666));
#12504=CARTESIAN_POINT('Ctrl Pts',(0.227319688237882,-1.18351239299796,
0.203150045648192));
#12505=CARTESIAN_POINT('Ctrl Pts',(0.237926932441998,-1.17293746916702,
0.405609838636422));
#12506=CARTESIAN_POINT('Ctrl Pts',(0.248534117816369,-1.1623628476683,0.608069650238703));
#12507=CARTESIAN_POINT('Ctrl Pts',(0.200219987929043,-1.14439035743082,
-0.00103956457010847));
#12508=CARTESIAN_POINT('Ctrl Pts',(0.210830491339948,-1.13382006821851,
0.201420337884579));
#12509=CARTESIAN_POINT('Ctrl Pts',(0.221440906577676,-1.12324995278282,
0.403880253819325));
#12510=CARTESIAN_POINT('Ctrl Pts',(0.232051411471599,-1.11268010558856,
0.606340179010355));
#12511=CARTESIAN_POINT('Ctrl Pts',(0.200161975173303,-1.12312592850316,
-0.00214651389202307));
#12512=CARTESIAN_POINT('Ctrl Pts',(0.210772455448684,-1.11255764422181,
0.200313510564959));
#12513=CARTESIAN_POINT('Ctrl Pts',(0.221382936352032,-1.1019895901204,0.402773547004277));
#12514=CARTESIAN_POINT('Ctrl Pts',(0.231993417893744,-1.09142177001972,
0.605233595624295));
#12515=CARTESIAN_POINT('Origin',(10.4681436286308,-1.08420482109828,0.6));
#12516=CARTESIAN_POINT('',(10.5680065821063,-1.08420482079361,0.605233595624295));
#12517=CARTESIAN_POINT('Origin',(10.4681436286308,-1.08420482099672,0.600000000000001));
#12518=CARTESIAN_POINT('Origin',(10.4681436286308,-1.08420482109828,0.6));
#12519=CARTESIAN_POINT('Origin',(10.4681436286308,0.7,0.6));
#12520=CARTESIAN_POINT('',(10.5680065821063,0.7,0.605233595624295));
#12521=CARTESIAN_POINT('Ctrl Pts',(10.599839982685,-1.11594741464673,-0.00218387205330164));
#12522=CARTESIAN_POINT('Ctrl Pts',(10.5892288496247,-1.10536637943871,0.200288608282177));
#12523=CARTESIAN_POINT('Ctrl Pts',(10.5786177161011,-1.0947855138519,0.402761097457634));
#12524=CARTESIAN_POINT('Ctrl Pts',(10.5680065821063,-1.08420482079362,0.605233595624295));
#12525=CARTESIAN_POINT('Ctrl Pts',(10.5997613205547,-1.14474784499259,-0.000682909193257743));
#12526=CARTESIAN_POINT('Ctrl Pts',(10.5891501209488,-1.13416481604349,0.201789447273867));
#12527=CARTESIAN_POINT('Ctrl Pts',(10.5785391399155,-1.12358205581644,0.404261829287571));
#12528=CARTESIAN_POINT('Ctrl Pts',(10.5679279386544,-1.11299934606825,0.606734202078189));
#12529=CARTESIAN_POINT('Ctrl Pts',(10.5764119435127,-1.19466846760808,0.000702210001053139));
#12530=CARTESIAN_POINT('Ctrl Pts',(10.5658041809617,-1.18408222297768,0.203174550667819));
#12531=CARTESIAN_POINT('Ctrl Pts',(10.5551963844732,-1.17349608774572,0.405646894856767));
#12532=CARTESIAN_POINT('Ctrl Pts',(10.544588659013,-1.16291012508165,0.608119251464957));
#12533=CARTESIAN_POINT('Ctrl Pts',(10.5269342003857,-1.21442651155969,-0.000858270497959616));
#12534=CARTESIAN_POINT('Ctrl Pts',(10.5163317654776,-1.20384274018949,0.201614467507756));
#12535=CARTESIAN_POINT('Ctrl Pts',(10.5057293269973,-1.1932591813998,0.404087216090532));
#12536=CARTESIAN_POINT('Ctrl Pts',(10.4951269905998,-1.18267571840064,0.606559974437339));
#12537=CARTESIAN_POINT('Ctrl Pts',(10.5053655128635,-1.21565094114741,-0.0019246498908503));
#12538=CARTESIAN_POINT('Ctrl Pts',(10.4947646468921,-1.20506932615592,0.200548282383137));
#12539=CARTESIAN_POINT('Ctrl Pts',(10.4841638390504,-1.19448787589602,0.403021225840181));
#12540=CARTESIAN_POINT('Ctrl Pts',(10.4735630903435,-1.18390659316268,0.605494180667945));
#12541=CARTESIAN_POINT('Ctrl Pts',(10.5997255308004,-1.11583328740478,1.02782365951626E-16));
#12542=CARTESIAN_POINT('Ctrl Pts',(10.589152548365,-1.10529029582828,0.201744523047832));
#12543=CARTESIAN_POINT('Ctrl Pts',(10.5785795654695,-1.09474747266587,0.40348905487273));
#12544=CARTESIAN_POINT('Ctrl Pts',(10.5680065821063,-1.08420482079362,0.605233595624295));
#12545=CARTESIAN_POINT('Ctrl Pts',(10.5053638082297,1.21564923960921,-0.0018920919656423));
#12546=CARTESIAN_POINT('Ctrl Pts',(10.4947635104759,1.20506819181477,0.200569987667808));
#12547=CARTESIAN_POINT('Ctrl Pts',(10.4841632708454,1.19448730873444,0.403032078483127));
#12548=CARTESIAN_POINT('Ctrl Pts',(10.4735630903435,1.18390659316268,0.605494180667945));
#12549=CARTESIAN_POINT('Ctrl Pts',(10.5341220579192,1.21401666636749,-0.000470252816738081));
#12550=CARTESIAN_POINT('Ctrl Pts',(10.5235196325477,1.20343268662274,0.201991562854702));
#12551=CARTESIAN_POINT('Ctrl Pts',(10.5129172908767,1.19284910679518,0.404453403808947));
#12552=CARTESIAN_POINT('Ctrl Pts',(10.5023149573519,1.18226542681329,0.606915239027137));
#12553=CARTESIAN_POINT('Ctrl Pts',(10.5827170203615,1.18801090922716,0.000717463067903341));
#12554=CARTESIAN_POINT('Ctrl Pts',(10.5721088691741,1.17742555398174,0.203178921531494));
#12555=CARTESIAN_POINT('Ctrl Pts',(10.5615007184277,1.16684027916303,0.405640383775807));
#12556=CARTESIAN_POINT('Ctrl Pts',(10.5508925935528,1.15625520969485,0.60810185787831));
#12557=CARTESIAN_POINT('Ctrl Pts',(10.5997792798033,1.13754603572512,-0.00102559206997387));
#12558=CARTESIAN_POINT('Ctrl Pts',(10.5891686973038,1.12696411138589,0.201435946515793));
#12559=CARTESIAN_POINT('Ctrl Pts',(10.5785581831385,1.11638231376635,0.40389749513889));
#12560=CARTESIAN_POINT('Ctrl Pts',(10.5679475995174,1.10580071474959,0.606359050464716));
#12561=CARTESIAN_POINT('Ctrl Pts',(10.5998382764002,1.11594571320176,-0.00215131420076595));
#12562=CARTESIAN_POINT('Ctrl Pts',(10.5892277121014,1.10536524516024,0.200310313518148));
#12563=CARTESIAN_POINT('Ctrl Pts',(10.5786171473394,1.09478494672192,0.402771950076102));
#12564=CARTESIAN_POINT('Ctrl Pts',(10.5680065821063,1.08420482079361,0.605233595624295));
#12565=CARTESIAN_POINT('Ctrl Pts',(10.5680065821063,1.08420482079361,0.605233595624295));
#12566=CARTESIAN_POINT('Ctrl Pts',(10.5785795654695,1.09474747266587,0.40348905487273));
#12567=CARTESIAN_POINT('Ctrl Pts',(10.589152548365,1.10529029582828,0.201744523047831));
#12568=CARTESIAN_POINT('Ctrl Pts',(10.5997255308004,1.11583328740478,1.07661275727811E-16));
#12569=CARTESIAN_POINT('Ctrl Pts',(10.1947388861048,1.09885088260187,0.7));
#12570=CARTESIAN_POINT('Ctrl Pts',(10.285877616441,1.09404209584202,0.7));
#12571=CARTESIAN_POINT('Ctrl Pts',(10.3770124662346,1.0891584122264,0.7));
#12572=CARTESIAN_POINT('Ctrl Pts',(10.4681436286308,1.08420482079361,0.7));
#12573=CARTESIAN_POINT('Ctrl Pts',(10.196260416419,1.12768774893097,0.700000000000001));
#12574=CARTESIAN_POINT('Ctrl Pts',(10.2874149314686,1.12287675076168,0.699999949550842));
#12575=CARTESIAN_POINT('Ctrl Pts',(10.3785648662465,1.11799094453753,0.700000051218742));
#12576=CARTESIAN_POINT('Ctrl Pts',(10.4697107510168,1.11303515260326,0.7));
#12577=CARTESIAN_POINT('Ctrl Pts',(10.1988975981852,1.17766904563614,0.67669140632491));
#12578=CARTESIAN_POINT('Ctrl Pts',(10.2900793016129,1.17285439035486,0.676693724638983));
#12579=CARTESIAN_POINT('Ctrl Pts',(10.3812557252598,1.16796482352885,0.676696026813929));
#12580=CARTESIAN_POINT('Ctrl Pts',(10.4724269697127,1.16300539549315,0.676698381019544));
#12581=CARTESIAN_POINT('Ctrl Pts',(10.1999375452555,1.19737868557977,0.627098033786781));
#12582=CARTESIAN_POINT('Ctrl Pts',(10.2911301919381,1.19256517083271,0.627104033151799));
#12583=CARTESIAN_POINT('Ctrl Pts',(10.382317043787,1.18767684023183,0.627110048826767));
#12584=CARTESIAN_POINT('Ctrl Pts',(10.4734985149421,1.18271860027509,0.627116141711795));
#12585=CARTESIAN_POINT('Ctrl Pts',(10.1999999975038,1.19856231440453,0.605472757505366));
#12586=CARTESIAN_POINT('Ctrl Pts',(10.2911933328565,1.19375025772558,0.605479840815741));
#12587=CARTESIAN_POINT('Ctrl Pts',(10.3823809652617,1.18886335120032,0.605486986548286));
#12588=CARTESIAN_POINT('Ctrl Pts',(10.4735630903435,1.18390659316268,0.605494180667944));
#12589=CARTESIAN_POINT('Ctrl Pts',(0.200159601751749,1.12312829248604,-0.00219180147311912));
#12590=CARTESIAN_POINT('Ctrl Pts',(0.210770873167554,1.11255922017607,0.200283318842441));
#12591=CARTESIAN_POINT('Ctrl Pts',(0.221382145211419,1.10199037808008,0.402758451142111));
#12592=CARTESIAN_POINT('Ctrl Pts',(0.231993417893744,1.09142177001972,0.605233595624295));
#12593=CARTESIAN_POINT('Ctrl Pts',(0.200236952094631,1.15148086499205,-0.000715869007730825));
#12594=CARTESIAN_POINT('Ctrl Pts',(0.210848310847714,1.14090905181173,0.201759082033021));
#12595=CARTESIAN_POINT('Ctrl Pts',(0.221459381762758,1.13033759660317,0.404234066901971));
#12596=CARTESIAN_POINT('Ctrl Pts',(0.232070742664217,1.11976621744484,0.606709040139042));
#12597=CARTESIAN_POINT('Ctrl Pts',(0.222806696702742,1.20067708175657,0.000669311976984441));
#12598=CARTESIAN_POINT('Ctrl Pts',(0.233413416075889,1.19010082554658,0.203144236955742));
#12599=CARTESIAN_POINT('Ctrl Pts',(0.244020198555212,1.17952469009474,0.405619164345205));
#12600=CARTESIAN_POINT('Ctrl Pts',(0.254626870458834,1.16894881850735,0.608094110943904));
#12601=CARTESIAN_POINT('Ctrl Pts',(0.271086891015657,1.22096622390789,-0.000801865493577694));
#12602=CARTESIAN_POINT('Ctrl Pts',(0.281686280594249,1.21039315447922,0.201673594461172));
#12603=CARTESIAN_POINT('Ctrl Pts',(0.292285672737775,1.1998203699977,0.404149068703718));
#12604=CARTESIAN_POINT('Ctrl Pts',(0.302884933932915,1.18924771644243,0.606624555877912));
#12605=CARTESIAN_POINT('Ctrl Pts',(0.292287201081515,1.22267118699778,-0.00182392867695869));
#12606=CARTESIAN_POINT('Ctrl Pts',(0.302884364349574,1.21210098433295,0.200651796350731));
#12607=CARTESIAN_POINT('Ctrl Pts',(0.313481451159089,1.20153100270242,0.403127536304793));
#12608=CARTESIAN_POINT('Ctrl Pts',(0.324078460244491,1.19096124572524,0.605603291426262));
#12609=CARTESIAN_POINT('Origin',(10.6002740930491,1.4,-0.0104671912485891));
#12610=CARTESIAN_POINT('Origin',(0.331856371369202,1.09142177001972,0.6));
#12611=CARTESIAN_POINT('',(0.3318563713692,1.09142177001972,0.9));
#12612=CARTESIAN_POINT('',(0.0322675109428288,1.09142177001972,0.615700786872883));
#12613=CARTESIAN_POINT('Origin',(0.3318563713692,1.09142177001972,0.6));
#12614=CARTESIAN_POINT('',(0.308522637995069,1.39004019713626,0.616809874278785));
#12615=CARTESIAN_POINT('Origin',(0.331856371369202,1.09142177001972,0.6));
#12616=CARTESIAN_POINT('Origin',(0.331856371369201,1.09142177001972,0.6));
#12617=CARTESIAN_POINT('Origin',(10.4681436286308,1.08420482079361,0.6));
#12618=CARTESIAN_POINT('',(10.4681436286308,1.08420482109828,0.9));
#12619=CARTESIAN_POINT('',(10.4844020137689,1.3833101379008,0.616482542003833));
#12620=CARTESIAN_POINT('Origin',(10.4681436258201,1.08420482094639,0.6));
#12621=CARTESIAN_POINT('',(10.7677324890572,1.08420482079361,0.615700786872884));
#12622=CARTESIAN_POINT('Origin',(10.4681436286308,1.08420482079361,0.6));
#12623=CARTESIAN_POINT('Origin',(10.4681436286308,1.08420482079362,0.6));
#12624=CARTESIAN_POINT('Origin',(0.3318563713692,-1.09142177001972,0.6));
#12625=CARTESIAN_POINT('',(0.3318563713692,-1.09142177001972,0.9));
#12626=CARTESIAN_POINT('',(0.308522637995069,-1.39004019713626,0.616809874278785));
#12627=CARTESIAN_POINT('Origin',(0.3318563713692,-1.09142177001972,0.6));
#12628=CARTESIAN_POINT('',(0.0322675109428289,-1.09142177001972,0.615700786872884));
#12629=CARTESIAN_POINT('Origin',(0.3318563713692,-1.09142177001972,0.6));
#12630=CARTESIAN_POINT('Origin',(0.331856371369201,-1.09142177001972,0.6));
#12631=CARTESIAN_POINT('Origin',(0.3318563713692,-0.7,0.6));
#12632=CARTESIAN_POINT('',(0.0322675109428288,-0.7,0.615700786872883));
#12633=CARTESIAN_POINT('',(0.3318563713692,-0.7,0.9));
#12634=CARTESIAN_POINT('Ctrl Pts',(0.276048389810261,-1.42252533450788,
-0.00533608639730399));
#12635=CARTESIAN_POINT('Ctrl Pts',(0.28687338241706,-1.4116967417008,0.202045878554724));
#12636=CARTESIAN_POINT('Ctrl Pts',(0.297698133178874,-1.40086836142621,
0.409427865329919));
#12637=CARTESIAN_POINT('Ctrl Pts',(0.308522637995069,-1.39004019713626,
0.616809874278785));
#12638=CARTESIAN_POINT('Ctrl Pts',(0.191246496057484,-1.41570630783033,
-0.00124775669238285));
#12639=CARTESIAN_POINT('Ctrl Pts',(0.202080757839133,-1.40486573978029,
0.206133102090467));
#12640=CARTESIAN_POINT('Ctrl Pts',(0.212914648880055,-1.39402634701096,
0.413514041581016));
#12641=CARTESIAN_POINT('Ctrl Pts',(0.223748532748767,-1.38318608000504,
0.620894932085382));
#12642=CARTESIAN_POINT('Ctrl Pts',(0.0492682973509243,-1.33685850703924,
0.00207719607616587));
#12643=CARTESIAN_POINT('Ctrl Pts',(0.0601266125734448,-1.32601270457081,
0.209456583216085));
#12644=CARTESIAN_POINT('Ctrl Pts',(0.0709850253737815,-1.3151666447344,
0.416835949794532));
#12645=CARTESIAN_POINT('Ctrl Pts',(0.0818432319483421,-1.30432109509162,
0.624215353109623));
#12646=CARTESIAN_POINT('Ctrl Pts',(-0.000163444061205068,-1.18769013309795,
-0.00311869847265479));
#12647=CARTESIAN_POINT('Ctrl Pts',(0.0107049555364969,-1.17685886333949,
0.204261034729081));
#12648=CARTESIAN_POINT('Ctrl Pts',(0.0215730900970294,-1.16602762920277,
0.411640782964944));
#12649=CARTESIAN_POINT('Ctrl Pts',(0.0324414916763936,-1.15519677672624,
0.619020537031064));
#12650=CARTESIAN_POINT('Ctrl Pts',(-0.00033748371827097,-1.12389640457412,
-0.0064395729582146));
#12651=CARTESIAN_POINT('Ctrl Pts',(0.0105308471731094,-1.11307128361434,
0.200940534347673));
#12652=CARTESIAN_POINT('Ctrl Pts',(0.0213991787230862,-1.10224640406117,
0.408320654220332));
#12653=CARTESIAN_POINT('Ctrl Pts',(0.0322675109428289,-1.09142177001972,
0.615700786872884));
#12654=CARTESIAN_POINT('Ctrl Pts',(0.27632692456468,-1.42224670711126,5.13911829758129E-17));
#12655=CARTESIAN_POINT('Ctrl Pts',(0.287059068122268,-1.41151099373342,
0.20560326985903));
#12656=CARTESIAN_POINT('Ctrl Pts',(0.297790973931072,-1.40077548928706,
0.411206561171438));
#12657=CARTESIAN_POINT('Ctrl Pts',(0.308522637995069,-1.39004019713626,
0.616809874278785));
#12658=CARTESIAN_POINT('Ctrl Pts',(0.0322675109428289,-1.09142177001972,
0.615700786872884));
#12659=CARTESIAN_POINT('Ctrl Pts',(0.0215116733095221,-1.10213436178043,
0.410467178800746));
#12660=CARTESIAN_POINT('Ctrl Pts',(0.0107558363321879,-1.11284719399673,
0.205233583245308));
#12661=CARTESIAN_POINT('Ctrl Pts',(1.76901136968166E-16,-1.12356026268968,
-7.45931094670027E-17));
#12662=CARTESIAN_POINT('Origin',(10.4681436286308,-1.08420482109828,0.6));
#12663=CARTESIAN_POINT('',(10.7677324890572,-1.08420482079361,0.615700786872884));
#12664=CARTESIAN_POINT('',(10.4844020137689,-1.3833101379008,0.616482542003833));
#12665=CARTESIAN_POINT('Origin',(10.4681436286308,-1.08420482079361,0.600000000000001));
#12666=CARTESIAN_POINT('',(10.4681436258201,-1.08420482094639,0.9));
#12667=CARTESIAN_POINT('Origin',(10.4681436286308,-1.08420482109828,0.6));
#12668=CARTESIAN_POINT('Origin',(10.4681436286308,-1.08420482079361,0.6));
#12669=CARTESIAN_POINT('Origin',(10.4681436286308,0.7,0.6));
#12670=CARTESIAN_POINT('',(10.7677324890572,0.7,0.615700786872884));
#12671=CARTESIAN_POINT('',(10.4681436286308,0.7,0.9));
#12672=CARTESIAN_POINT('Ctrl Pts',(10.4681436286308,-1.08420482079361,0.9));
#12673=CARTESIAN_POINT('Ctrl Pts',(9.02115959826777,-1.16285813221549,0.9));
#12674=CARTESIAN_POINT('Ctrl Pts',(5.64262097844114,-1.30550334054488,0.9));
#12675=CARTESIAN_POINT('Ctrl Pts',(2.25816172369615,-1.24194126716656,0.9));
#12676=CARTESIAN_POINT('Ctrl Pts',(0.331856371369198,-1.09142177001972,
0.9));
#12677=CARTESIAN_POINT('Ctrl Pts',(10.4728449957889,-1.17069581622255,0.9));
#12678=CARTESIAN_POINT('Ctrl Pts',(9.02515960257209,-1.24945398332951,0.900002463983243));
#12679=CARTESIAN_POINT('Ctrl Pts',(5.64406008560805,-1.39235654229312,0.899995181674544));
#12680=CARTESIAN_POINT('Ctrl Pts',(2.25481214769604,-1.3286896492945,0.900006992415263));
#12681=CARTESIAN_POINT('Ctrl Pts',(0.325113511056834,-1.17771496230318,
0.9));
#12682=CARTESIAN_POINT('Ctrl Pts',(10.4809942371438,-1.32061731204901,0.830050158657121));
#12683=CARTESIAN_POINT('Ctrl Pts',(9.03210079995546,-1.3995487214628,0.829938185878055));
#12684=CARTESIAN_POINT('Ctrl Pts',(5.64656962219688,-1.54290142969263,0.82970437227026));
#12685=CARTESIAN_POINT('Ctrl Pts',(2.24896854757963,-1.47903552984056,0.829838703712927));
#12686=CARTESIAN_POINT('Ctrl Pts',(0.313425270489114,-1.32729771265557,
0.830156825336737));
#12687=CARTESIAN_POINT('Ctrl Pts',(10.4842082875648,-1.37974615923803,0.681348425135383));
#12688=CARTESIAN_POINT('Ctrl Pts',(9.03482793853036,-1.45862084618981,0.681058092399338));
#12689=CARTESIAN_POINT('Ctrl Pts',(5.64753778607331,-1.60187726023264,0.68045297450285));
#12690=CARTESIAN_POINT('Ctrl Pts',(2.24670449952385,-1.53809938127555,0.680799765935021));
#12691=CARTESIAN_POINT('Ctrl Pts',(0.308806004580392,-1.38641375285276,
0.681625057916928));
#12692=CARTESIAN_POINT('Ctrl Pts',(10.4844020137689,-1.3833101379008,0.616482542003833));
#12693=CARTESIAN_POINT('Ctrl Pts',(9.03499042108131,-1.46211428773623,0.616139856494792));
#12694=CARTESIAN_POINT('Ctrl Pts',(5.64759185703765,-1.60522711936681,0.615422163720642));
#12695=CARTESIAN_POINT('Ctrl Pts',(2.24657199659733,-1.54153220865049,0.615835494619844));
#12696=CARTESIAN_POINT('Ctrl Pts',(0.308522637995066,-1.39004019713626,
0.616809874278785));
#12697=CARTESIAN_POINT('Ctrl Pts',(0.308522637995066,-1.39004019713626,
0.616809874278785));
#12698=CARTESIAN_POINT('Ctrl Pts',(2.24657199659733,-1.54153220865049,0.615835494619844));
#12699=CARTESIAN_POINT('Ctrl Pts',(5.64759185703765,-1.60522711936681,0.615422163720642));
#12700=CARTESIAN_POINT('Ctrl Pts',(9.03499042108131,-1.46211428773623,0.616139856494792));
#12701=CARTESIAN_POINT('Ctrl Pts',(10.4844020137689,-1.3833101379008,0.616482542003833));
#12702=CARTESIAN_POINT('Ctrl Pts',(10.4681436258201,-1.08420482094639,0.900000000000001));
#12703=CARTESIAN_POINT('Ctrl Pts',(9.02115959639274,-1.16285813229465,0.9));
#12704=CARTESIAN_POINT('Ctrl Pts',(5.64262097750198,-1.30550334052724,0.9));
#12705=CARTESIAN_POINT('Ctrl Pts',(2.25816172369615,-1.24194126716656,0.9));
#12706=CARTESIAN_POINT('Ctrl Pts',(0.331856371369198,-1.09142177001972,
0.9));
#12707=CARTESIAN_POINT('Ctrl Pts',(10.8003433549902,-1.11672267507076,-0.00655160349952438));
#12708=CARTESIAN_POINT('Ctrl Pts',(10.7894730668347,-1.10588321133639,0.200865850630566));
#12709=CARTESIAN_POINT('Ctrl Pts',(10.7786027781932,-1.09504392553578,0.408283314033857));
#12710=CARTESIAN_POINT('Ctrl Pts',(10.7677324890572,-1.08420482079361,0.615700786872885));
#12711=CARTESIAN_POINT('Ctrl Pts',(10.8001073672393,-1.20312439623403,-0.00204868896805508));
#12712=CARTESIAN_POINT('Ctrl Pts',(10.7892368724076,-1.19227880391739,0.205368384315645));
#12713=CARTESIAN_POINT('Ctrl Pts',(10.7783670568079,-1.18143370221047,0.41278551899075));
#12714=CARTESIAN_POINT('Ctrl Pts',(10.7674965587017,-1.17058839661753,0.620202606234566));
#12715=CARTESIAN_POINT('Ctrl Pts',(10.7300137544668,-1.35289768637741,0.00210488808650419));
#12716=CARTESIAN_POINT('Ctrl Pts',(10.7191538066016,-1.34204221082848,0.209521911971666));
#12717=CARTESIAN_POINT('Ctrl Pts',(10.7082938463195,-1.33118673671862,0.416938933985702));
#12718=CARTESIAN_POINT('Ctrl Pts',(10.6974340169938,-1.32033143065575,0.624355970618915));
#12719=CARTESIAN_POINT('Ctrl Pts',(10.5816241002662,-1.4121605627967,-0.00257485550010117));
#12720=CARTESIAN_POINT('Ctrl Pts',(10.5707805459565,-1.4013126969686,0.204843391064434));
#12721=CARTESIAN_POINT('Ctrl Pts',(10.5599369567012,-1.39046512672587,0.412261650129749));
#12722=CARTESIAN_POINT('Ctrl Pts',(10.5490937145378,-1.37961751361469,0.619679923312015));
#12723=CARTESIAN_POINT('Ctrl Pts',(10.5169176890673,-1.41583338198674,-0.00577403633861717));
#12724=CARTESIAN_POINT('Ctrl Pts',(10.5060789456421,-1.40499213715574,0.201644806368331));
#12725=CARTESIAN_POINT('Ctrl Pts',(10.4952403861233,-1.39415105487295,0.40906366572247));
#12726=CARTESIAN_POINT('Ctrl Pts',(10.4844020137689,-1.3833101379008,0.616482542003833));
#12727=CARTESIAN_POINT('Ctrl Pts',(10.8,-1.11638029377732,-2.51534904016637E-17));
#12728=CARTESIAN_POINT('Ctrl Pts',(10.7892441634977,-1.10565496086826,0.205233586491178));
#12729=CARTESIAN_POINT('Ctrl Pts',(10.7784883265195,-1.09492980219801,0.410467182062988));
#12730=CARTESIAN_POINT('Ctrl Pts',(10.7677324890572,-1.08420482079361,0.615700786872885));
#12731=CARTESIAN_POINT('Ctrl Pts',(10.4844020137689,-1.3833101379008,0.616482542003833));
#12732=CARTESIAN_POINT('Ctrl Pts',(10.4951398148107,-1.39405045994841,0.410988344812119));
#12733=CARTESIAN_POINT('Ctrl Pts',(10.5058777995597,-1.40479094425298,0.205494164234945));
#12734=CARTESIAN_POINT('Ctrl Pts',(10.5166159648474,-1.4155315881283,-2.5652223401007E-16));
#12735=CARTESIAN_POINT('Ctrl Pts',(10.5169125872774,1.41582827901939,-0.0056764044152427));
#12736=CARTESIAN_POINT('Ctrl Pts',(10.5060755445066,1.40498873522851,0.20170989432247));
#12737=CARTESIAN_POINT('Ctrl Pts',(10.4952386855848,1.39414935393528,0.409096209702196));
#12738=CARTESIAN_POINT('Ctrl Pts',(10.4844020137689,1.3833101379008,0.616482542003833));
#12739=CARTESIAN_POINT('Ctrl Pts',(10.6031877991504,1.41093118264609,-0.00141083033817288));
#12740=CARTESIAN_POINT('Ctrl Pts',(10.5923442181457,1.40008262840665,0.205974657203891));
#12741=CARTESIAN_POINT('Ctrl Pts',(10.5815009048179,1.38923496752292,0.413360205434192));
#12742=CARTESIAN_POINT('Ctrl Pts',(10.5706576147941,1.37838663885266,0.62074571708141));
#12743=CARTESIAN_POINT('Ctrl Pts',(10.7489822201969,1.33286898269122,0.00215046584238339));
#12744=CARTESIAN_POINT('Ctrl Pts',(10.7381210493968,1.32201618867047,0.209534855263179));
#12745=CARTESIAN_POINT('Ctrl Pts',(10.7272598662103,1.31116338896628,0.416919242515175));
#12746=CARTESIAN_POINT('Ctrl Pts',(10.716398780155,1.30031077634578,0.624303643734563));
#12747=CARTESIAN_POINT('Ctrl Pts',(10.8001612475457,1.18151886169146,-0.00307678645922502));
#12748=CARTESIAN_POINT('Ctrl Pts',(10.7892926103682,1.17067663552019,0.20430785074418));
#12749=CARTESIAN_POINT('Ctrl Pts',(10.7784241800195,1.15983442267521,0.41169249890798));
#12750=CARTESIAN_POINT('Ctrl Pts',(10.7675555412906,1.14899250266155,0.619077151394146));
#12751=CARTESIAN_POINT('Ctrl Pts',(10.8003382383521,1.11671757294177,-0.00645397222975308));
#12752=CARTESIAN_POINT('Ctrl Pts',(10.7894696557425,1.1058798099729,0.200930938146656));
#12753=CARTESIAN_POINT('Ctrl Pts',(10.778601072647,1.09504222488243,0.408315857793383));
#12754=CARTESIAN_POINT('Ctrl Pts',(10.7677324890572,1.08420482079361,0.615700786872884));
#12755=CARTESIAN_POINT('Ctrl Pts',(10.5166159648474,1.4155315881283,3.37837396946483E-16));
#12756=CARTESIAN_POINT('Ctrl Pts',(10.5058777995597,1.40479094425298,0.205494164234944));
#12757=CARTESIAN_POINT('Ctrl Pts',(10.4951398148107,1.39405045994841,0.41098834481212));
#12758=CARTESIAN_POINT('Ctrl Pts',(10.4844020137689,1.3833101379008,0.616482542003833));
#12759=CARTESIAN_POINT('Ctrl Pts',(10.7677324890572,1.08420482079361,0.615700786872884));
#12760=CARTESIAN_POINT('Ctrl Pts',(10.7784883265195,1.09492980219801,0.410467182062988));
#12761=CARTESIAN_POINT('Ctrl Pts',(10.7892441634977,1.10565496086826,0.205233586491177));
#12762=CARTESIAN_POINT('Ctrl Pts',(10.8,1.11638029377732,-4.7271214720368E-17));
#12763=CARTESIAN_POINT('Ctrl Pts',(0.3318563713692,1.09142177001972,0.9));
#12764=CARTESIAN_POINT('Ctrl Pts',(1.77658538561441,1.20431139287985,0.9));
#12765=CARTESIAN_POINT('Ctrl Pts',(5.15852145577913,1.31798734362749,0.900000000000001));
#12766=CARTESIAN_POINT('Ctrl Pts',(8.53883158814675,1.18907590268945,0.9));
#12767=CARTESIAN_POINT('Ctrl Pts',(10.4681436286308,1.08420482079361,0.9));
#12768=CARTESIAN_POINT('Ctrl Pts',(0.325113511056836,1.17771496230318,0.9));
#12769=CARTESIAN_POINT('Ctrl Pts',(1.77238748853623,1.29094597754667,0.900005244311447));
#12770=CARTESIAN_POINT('Ctrl Pts',(5.15940689953628,1.40489117512763,0.899995532233175));
#12771=CARTESIAN_POINT('Ctrl Pts',(8.54259780483314,1.2757067056985,0.90000328531099));
#12772=CARTESIAN_POINT('Ctrl Pts',(10.4728449957889,1.17069581622255,0.9));
#12773=CARTESIAN_POINT('Ctrl Pts',(0.313425270489116,1.32729771265557,0.830156825336737));
#12774=CARTESIAN_POINT('Ctrl Pts',(1.76508272830699,1.44110107554431,0.829918234118879));
#12775=CARTESIAN_POINT('Ctrl Pts',(5.16095094050242,1.55552201031752,0.829677185710002));
#12776=CARTESIAN_POINT('Ctrl Pts',(8.54913632089268,1.4258591912674,0.829900861618366));
#12777=CARTESIAN_POINT('Ctrl Pts',(10.4809942371438,1.32061731204901,0.830050158657121));
#12778=CARTESIAN_POINT('Ctrl Pts',(0.308806004580394,1.38641375285276,0.681625057916928));
#12779=CARTESIAN_POINT('Ctrl Pts',(1.76222987578798,1.50017797416985,0.681006088930498));
#12780=CARTESIAN_POINT('Ctrl Pts',(5.16154986224672,1.61450132085358,0.68038246417749));
#12781=CARTESIAN_POINT('Ctrl Pts',(8.55170115551887,1.48491240850707,0.680961314820656));
#12782=CARTESIAN_POINT('Ctrl Pts',(10.4842082875648,1.37974615923803,0.681348425135383));
#12783=CARTESIAN_POINT('Ctrl Pts',(0.308522637995068,1.39004019713626,0.616809874278785));
#12784=CARTESIAN_POINT('Ctrl Pts',(1.76205965694675,1.50365920577193,0.616079089534579));
#12785=CARTESIAN_POINT('Ctrl Pts',(5.16158497046229,1.61783515152865,0.615338844765104));
#12786=CARTESIAN_POINT('Ctrl Pts',(8.55185322351876,1.48838233768137,0.616025627991778));
#12787=CARTESIAN_POINT('Ctrl Pts',(10.4844020137689,1.3833101379008,0.616482542003833));
#12788=CARTESIAN_POINT('Ctrl Pts',(10.4844020137689,1.3833101379008,0.616482542003833));
#12789=CARTESIAN_POINT('Ctrl Pts',(8.55185322351876,1.48838233768137,0.616025627991778));
#12790=CARTESIAN_POINT('Ctrl Pts',(5.16158497046229,1.61783515152865,0.615338844765104));
#12791=CARTESIAN_POINT('Ctrl Pts',(1.76205965694675,1.50365920577193,0.616079089534579));
#12792=CARTESIAN_POINT('Ctrl Pts',(0.308522637995068,1.39004019713626,0.616809874278785));
#12793=CARTESIAN_POINT('Ctrl Pts',(0.3318563713692,1.09142177001972,0.9));
#12794=CARTESIAN_POINT('Ctrl Pts',(1.77658538561441,1.20431139287985,0.9));
#12795=CARTESIAN_POINT('Ctrl Pts',(5.15852145577913,1.31798734362749,0.900000000000001));
#12796=CARTESIAN_POINT('Ctrl Pts',(8.53883158814675,1.18907590268945,0.9));
#12797=CARTESIAN_POINT('Ctrl Pts',(10.4681436286308,1.08420482079361,0.9));
#12798=CARTESIAN_POINT('Ctrl Pts',(-0.000344602063817145,1.12390349461883,
-0.00657539908256866));
#12799=CARTESIAN_POINT('Ctrl Pts',(0.0105261016091243,1.11307601020539,
0.200849983592616));
#12800=CARTESIAN_POINT('Ctrl Pts',(0.0213968059409475,1.10224876730309,
0.408275378840013));
#12801=CARTESIAN_POINT('Ctrl Pts',(0.0322675109428289,1.09142177001972,
0.615700786872884));
#12802=CARTESIAN_POINT('Ctrl Pts',(-0.000112549170678945,1.2089618047365,
-0.00214756610981592));
#12803=CARTESIAN_POINT('Ctrl Pts',(0.0107584275574203,1.19812589474889,
0.205277296000037));
#12804=CARTESIAN_POINT('Ctrl Pts',(0.021628504370896,1.18729063034778,0.412702239156743));
#12805=CARTESIAN_POINT('Ctrl Pts',(0.0324994852542487,1.17645511229507,
0.620127120417125));
#12806=CARTESIAN_POINT('Ctrl Pts',(0.0675181008536004,1.35659180908255,
0.00201426213057289));
#12807=CARTESIAN_POINT('Ctrl Pts',(0.0783748317004002,1.34574224493831,
0.20943904356877));
#12808=CARTESIAN_POINT('Ctrl Pts',(0.0892318011706237,1.33489254525337,
0.416863803530356));
#12809=CARTESIAN_POINT('Ctrl Pts',(0.100088380073201,1.32404321751407,0.624288602298589));
#12810=CARTESIAN_POINT('Ctrl Pts',(0.212439875011655,1.41741816253371,-0.00240566592686199));
#12811=CARTESIAN_POINT('Ctrl Pts',(0.223274062163905,1.40657840226088,0.20502076110302));
#12812=CARTESIAN_POINT('Ctrl Pts',(0.234108278795672,1.39573903465802,0.412447205628077));
#12813=CARTESIAN_POINT('Ctrl Pts',(0.244942059060342,1.38489960928785,0.619873667633733));
#12814=CARTESIAN_POINT('Ctrl Pts',(0.276041299849618,1.42253242682652,-0.00547191373834488));
#12815=CARTESIAN_POINT('Ctrl Pts',(0.286868655882245,1.41170146982041,0.201955326984501));
#12816=CARTESIAN_POINT('Ctrl Pts',(0.297695769965166,1.40087072543886,0.409382589539965));
#12817=CARTESIAN_POINT('Ctrl Pts',(0.308522637995069,1.39004019713626,0.616809874278785));
#12818=CARTESIAN_POINT('Ctrl Pts',(2.26869304592592E-17,1.12356026268968,
-3.16587034365767E-17));
#12819=CARTESIAN_POINT('Ctrl Pts',(0.0107558363321878,1.11284719399672,
0.205233583245308));
#12820=CARTESIAN_POINT('Ctrl Pts',(0.0215116733095221,1.10213436178043,
0.410467178800746));
#12821=CARTESIAN_POINT('Ctrl Pts',(0.0322675109428289,1.09142177001972,
0.615700786872884));
#12822=CARTESIAN_POINT('Ctrl Pts',(0.308522637995069,1.39004019713626,0.616809874278785));
#12823=CARTESIAN_POINT('Ctrl Pts',(0.297790973931072,1.40077548928706,0.411206561171438));
#12824=CARTESIAN_POINT('Ctrl Pts',(0.287059068122271,1.41151099373341,0.205603269859031));
#12825=CARTESIAN_POINT('Ctrl Pts',(0.276326924564681,1.42224670711126,-2.68882138776405E-16));
#12826=CARTESIAN_POINT('Ctrl Pts',(10.5166159648474,-1.4155315881283,0.));
#12827=CARTESIAN_POINT('Ctrl Pts',(10.5064062201588,-1.40475637621136,0.205603291426271));
#12828=CARTESIAN_POINT('Ctrl Pts',(10.4961964754701,-1.39398116429443,0.411206582852543));
#12829=CARTESIAN_POINT('Ctrl Pts',(10.4859867307814,-1.38320595237749,0.616809874278814));
#12830=CARTESIAN_POINT('Ctrl Pts',(7.10318628475318,-1.599994843061,0.));
#12831=CARTESIAN_POINT('Ctrl Pts',(7.09978773046573,-1.58921963114407,0.205603291426271));
#12832=CARTESIAN_POINT('Ctrl Pts',(7.09638917617828,-1.57844441922713,0.411206582852543));
#12833=CARTESIAN_POINT('Ctrl Pts',(7.09299062189083,-1.5676692073102,0.616809874278814));
#12834=CARTESIAN_POINT('Ctrl Pts',(3.68975660465893,-1.68747752195839,0.));
#12835=CARTESIAN_POINT('Ctrl Pts',(3.69316924077269,-1.67670231004145,0.205603291426272));
#12836=CARTESIAN_POINT('Ctrl Pts',(3.69658187688646,-1.66592709812452,0.411206582852543));
#12837=CARTESIAN_POINT('Ctrl Pts',(3.69999451300023,-1.65515188620758,0.616809874278814));
#12838=CARTESIAN_POINT('Ctrl Pts',(0.276326924564679,-1.42224670711126,
0.));
#12839=CARTESIAN_POINT('Ctrl Pts',(0.286550751079662,-1.41147149519433,
0.205603291426271));
#12840=CARTESIAN_POINT('Ctrl Pts',(0.296774577594646,-1.40069628327739,
0.411206582852543));
#12841=CARTESIAN_POINT('Ctrl Pts',(0.306998404109629,-1.38992107136046,
0.616809874278814));
#12842=CARTESIAN_POINT('Origin',(0.,-1.4,0.));
#12843=CARTESIAN_POINT('Origin',(5.4,-8.13935059369636E-18,0.9));
#12844=CARTESIAN_POINT('Ctrl Pts',(0.276326924564679,1.42224670711126,0.));
#12845=CARTESIAN_POINT('Ctrl Pts',(0.286550751079662,1.41147149519433,0.205603291426271));
#12846=CARTESIAN_POINT('Ctrl Pts',(0.296774577594645,1.40069628327739,0.411206582852543));
#12847=CARTESIAN_POINT('Ctrl Pts',(0.306998404109628,1.38992107136046,0.616809874278814));
#12848=CARTESIAN_POINT('Ctrl Pts',(3.68975660465893,1.68747752195839,0.));
#12849=CARTESIAN_POINT('Ctrl Pts',(3.6931692407727,1.67670231004145,0.205603291426271));
#12850=CARTESIAN_POINT('Ctrl Pts',(3.69658187688646,1.66592709812452,0.411206582852543));
#12851=CARTESIAN_POINT('Ctrl Pts',(3.69999451300023,1.65515188620758,0.616809874278814));
#12852=CARTESIAN_POINT('Ctrl Pts',(7.10318628475318,1.599994843061,0.));
#12853=CARTESIAN_POINT('Ctrl Pts',(7.09978773046573,1.58921963114407,0.205603291426271));
#12854=CARTESIAN_POINT('Ctrl Pts',(7.09638917617828,1.57844441922713,0.411206582852543));
#12855=CARTESIAN_POINT('Ctrl Pts',(7.09299062189083,1.5676692073102,0.616809874278814));
#12856=CARTESIAN_POINT('Ctrl Pts',(10.5166159648474,1.4155315881283,0.));
#12857=CARTESIAN_POINT('Ctrl Pts',(10.5064062201588,1.40475637621136,0.205603291426271));
#12858=CARTESIAN_POINT('Ctrl Pts',(10.4961964754701,1.39398116429443,0.411206582852543));
#12859=CARTESIAN_POINT('Ctrl Pts',(10.4859867307814,1.38320595237749,0.616809874278814));
#12860=CARTESIAN_POINT('Origin',(10.8,1.4,0.));
#18563=UNCERTAINTY_MEASURE_WITH_UNIT(LENGTH_MEASURE(0.001),#18581,
'DISTANCE_ACCURACY_VALUE',
'Maximum model space distance between geometric entities at asserted c
onnectivities');
#18568=UNCERTAINTY_MEASURE_WITH_UNIT(LENGTH_MEASURE(0.001),#18581,
'DISTANCE_ACCURACY_VALUE',
'Maximum model space distance between geometric entities at asserted c
onnectivities');
#18575=(
GEOMETRIC_REPRESENTATION_CONTEXT(3)
GLOBAL_UNCERTAINTY_ASSIGNED_CONTEXT((#18563))
GLOBAL_UNIT_ASSIGNED_CONTEXT((#18581,#18583,#18584))
REPRESENTATION_CONTEXT('','3D')
);
#18580=(
GEOMETRIC_REPRESENTATION_CONTEXT(3)
GLOBAL_UNCERTAINTY_ASSIGNED_CONTEXT((#18568))
GLOBAL_UNIT_ASSIGNED_CONTEXT((#18581,#18583,#18584))
REPRESENTATION_CONTEXT('','3D')
);
#18581=(
LENGTH_UNIT()
NAMED_UNIT(*)
SI_UNIT(.CENTI.,.METRE.)
);
#18583=(
NAMED_UNIT(*)
PLANE_ANGLE_UNIT()
SI_UNIT($,.RADIAN.)
);
#18584=(
NAMED_UNIT(*)
SI_UNIT($,.STERADIAN.)
SOLID_ANGLE_UNIT()
);
#18591=SHAPE_DEFINITION_REPRESENTATION(#18602,#18629);
#18602=PRODUCT_DEFINITION_SHAPE('',$,#18641);
#18629=SHAPE_REPRESENTATION('',(#6832),#18575);
#18634=PRODUCT_DEFINITION_CONTEXT('part definition',#18669,'design');
#18641=PRODUCT_DEFINITION('2026-11-10-05-09-36-729',
'Lower structural shell',#18652,#18634);
#18652=PRODUCT_DEFINITION_FORMATION('',$,#18677);
#18669=APPLICATION_CONTEXT(
'Core Data for Automotive Mechanical Design Process');
#18670=PRODUCT_CONTEXT('part definition',#18669,'mechanical');
#18677=PRODUCT('2026-11-10-05-09-36-729','Lower structural shell',$,(#18670));
#18686=PRESENTATION_STYLE_ASSIGNMENT((#18694));
#18694=SURFACE_STYLE_USAGE(.BOTH.,#18702);
#18702=SURFACE_SIDE_STYLE('',(#18710));
#18710=SURFACE_STYLE_FILL_AREA(#18718);
#18718=FILL_AREA_STYLE('Structural dark blue',(#18726));
#18726=FILL_AREA_STYLE_COLOUR('Structural dark blue',#18734);
#18734=COLOUR_RGB('Structural dark blue',0.0901960784313725,0.270588235294118,
0.513725490196078);
ENDSEC;
END-ISO-10303-21;
